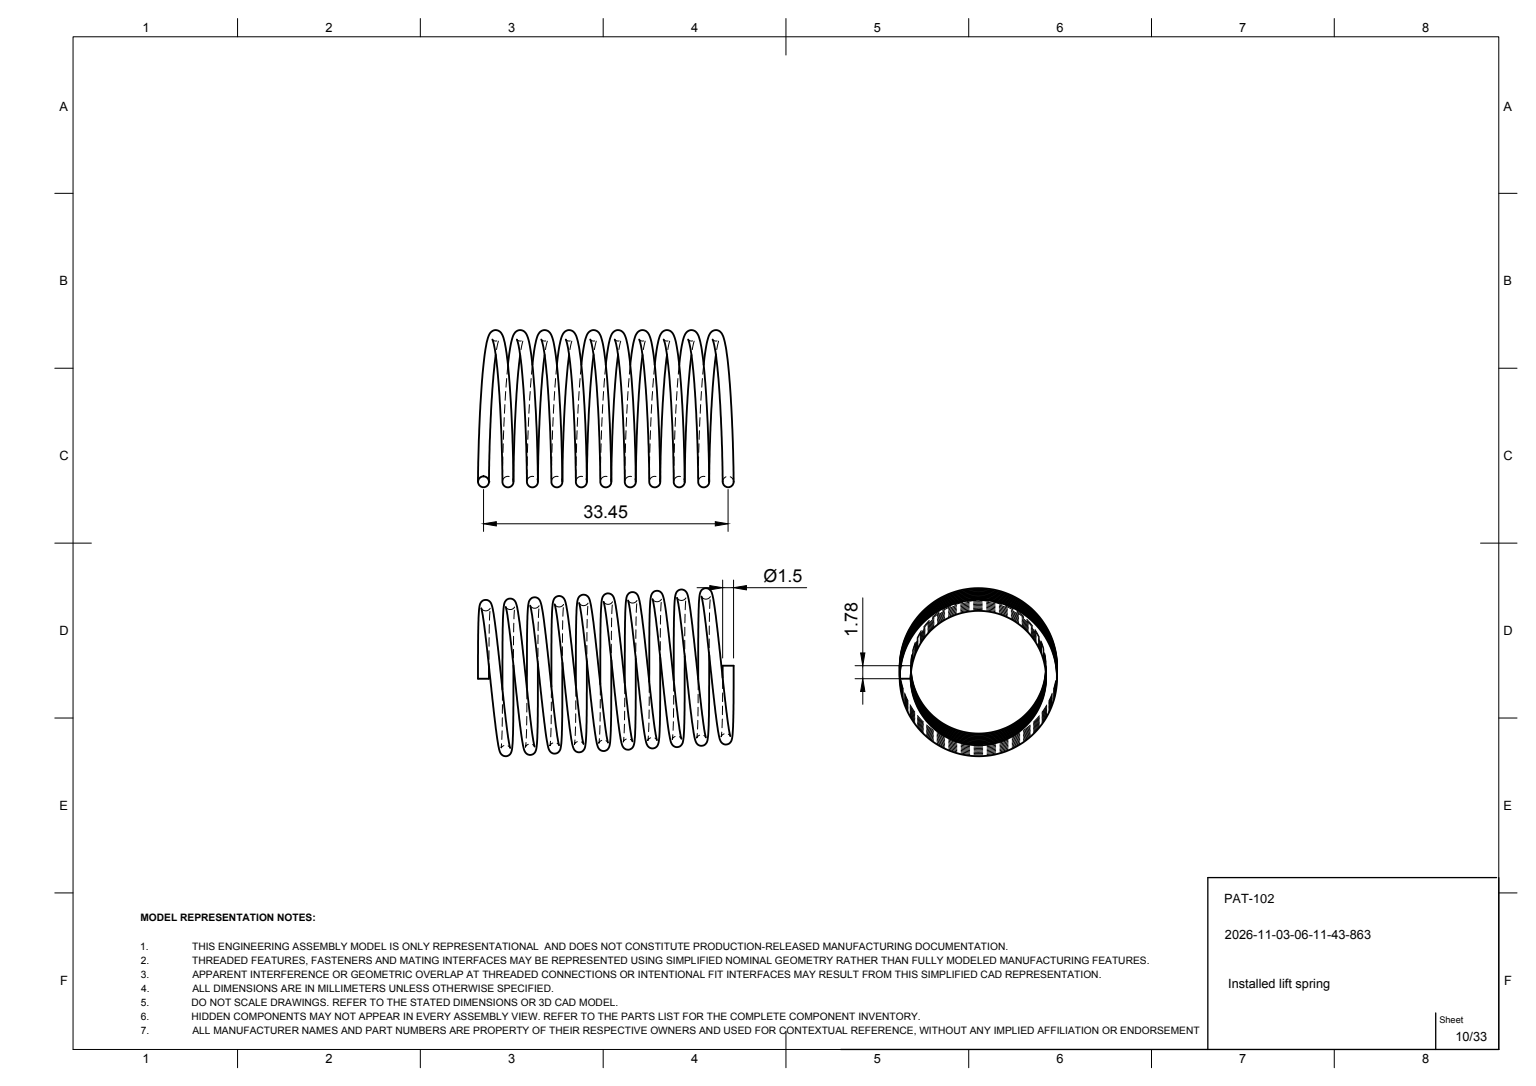
ISO-10303-21;
HEADER;
/* Generated by software containing ST-Developer
 * from STEP Tools, Inc. (www.steptools.com) 
 */

FILE_DESCRIPTION(
/* description */ ('Swing-away clamp arm'),
/* implementation_level */ '2;1');

FILE_NAME(
/* name */ 'Installed lift spring.step',
/* time_stamp */ '2026-10-28T03:26:03-07:00',
/* author */ (''),
/* organization */ (''),
/* preprocessor_version */ 'ST-DEVELOPER v20.2',
/* originating_system */ 'Autodesk Translation Framework v15.17.0.0',
/* authorisation */ '');

FILE_SCHEMA (('AUTOMOTIVE_DESIGN { 1 0 10303 214 3 1 1 }'));
ENDSEC;

DATA;
#10=MECHANICAL_DESIGN_GEOMETRIC_PRESENTATION_REPRESENTATION('',(#298),#10627);
#221=B_SPLINE_CURVE_WITH_KNOTS('',3,(#9145,#9146,#9147,#9148,#9149,#9150,
#9151,#9152,#9153,#9154,#9155,#9156,#9157,#9158,#9159,#9160,#9161,#9162,
#9163,#9164,#9165,#9166,#9167,#9168,#9169,#9170,#9171,#9172,#9173,#9174,
#9175,#9176,#9177,#9178,#9179,#9180,#9181,#9182,#9183,#9184,#9185,#9186,
#9187,#9188,#9189,#9190,#9191,#9192,#9193,#9194,#9195,#9196,#9197,#9198,
#9199,#9200,#9201,#9202,#9203,#9204,#9205,#9206,#9207,#9208,#9209,#9210,
#9211,#9212,#9213,#9214,#9215,#9216,#9217,#9218,#9219,#9220,#9221,#9222,
#9223,#9224,#9225,#9226,#9227,#9228,#9229,#9230,#9231,#9232,#9233,#9234,
#9235,#9236,#9237,#9238,#9239,#9240,#9241,#9242,#9243,#9244,#9245,#9246,
#9247,#9248,#9249,#9250,#9251,#9252,#9253,#9254,#9255,#9256,#9257,#9258,
#9259,#9260,#9261,#9262,#9263,#9264,#9265,#9266),.UNSPECIFIED.,.F.,.F.,
(4,1,1,1,1,1,1,1,1,1,1,1,1,1,1,1,1,1,1,1,1,1,1,1,1,1,1,1,1,1,1,1,1,1,1,
1,1,1,1,1,1,1,1,1,1,1,1,1,1,1,1,1,1,1,1,1,1,1,1,1,1,1,1,1,1,1,1,1,1,1,1,
1,1,1,1,1,1,1,1,1,1,1,1,1,1,1,1,1,1,1,1,1,1,1,1,1,1,1,1,1,1,1,1,1,1,1,1,
1,1,1,1,1,1,1,1,1,1,1,1,4),(0.,0.00892857142857143,0.0178571428571429,0.0267857142857143,
0.0357142857142857,0.0446428571428571,0.0535714285714286,0.0625,0.0714285714285714,
0.0803571428571428,0.0892857142857143,0.0982142857142857,0.107142857142857,
0.116071428571429,0.120535714285714,0.125,0.129464285714286,0.133928571428571,
0.138392857142857,0.142857142857143,0.150793650793651,0.154761904761905,
0.158730158730159,0.166666666666667,0.174603174603175,0.17989417989418,
0.19047619047619,0.198412698412698,0.206349206349206,0.214285714285714,
0.222222222222222,0.227513227513228,0.238095238095238,0.25,0.261904761904762,
0.273809523809524,0.285714285714286,0.297619047619048,0.30952380952381,
0.321428571428571,0.333333333333333,0.341269841269841,0.349206349206349,
0.357142857142857,0.365079365079365,0.37037037037037,0.380952380952381,
0.386243386243386,0.396825396825397,0.404761904761905,0.412698412698413,
0.420634920634921,0.428571428571429,0.44047619047619,0.452380952380952,
0.458333333333333,0.464285714285714,0.470238095238095,0.476190476190476,
0.484126984126984,0.492063492063492,0.5,0.502232142857143,0.504464285714286,
0.508928571428571,0.517857142857143,0.526785714285714,0.535714285714286,
0.544642857142857,0.553571428571429,0.5625,0.571428571428571,0.580357142857143,
0.589285714285714,0.598214285714286,0.607142857142857,0.616071428571429,
0.625,0.633928571428571,0.642857142857143,0.650793650793651,0.658730158730159,
0.666666666666667,0.678571428571428,0.69047619047619,0.702380952380952,
0.714285714285714,0.726190476190476,0.738095238095238,0.746031746031746,
0.753968253968254,0.761904761904762,0.76984126984127,0.777777777777778,
0.785714285714286,0.790178571428571,0.794642857142857,0.803571428571428,
0.8125,0.821428571428571,0.830357142857143,0.839285714285714,0.848214285714286,
0.857142857142857,0.866071428571429,0.875,0.883928571428571,0.892857142857143,
0.901785714285714,0.910714285714286,0.919642857142857,0.928571428571429,
0.9375,0.946428571428571,0.955357142857143,0.964285714285714,0.973214285714286,
0.982142857142857,0.991071428571429,1.),.UNSPECIFIED.);
#240=B_SPLINE_SURFACE_WITH_KNOTS('',3,3,((#7922,#7923,#7924,#7925,#7926,
#7927,#7928,#7929,#7930,#7931,#7932,#7933,#7934,#7935,#7936,#7937,#7938,
#7939,#7940,#7941,#7942,#7943,#7944,#7945,#7946,#7947,#7948,#7949,#7950,
#7951,#7952,#7953,#7954,#7955,#7956,#7957,#7958,#7959,#7960,#7961,#7962,
#7963,#7964,#7965,#7966,#7967,#7968,#7969,#7970,#7971,#7972,#7973,#7974,
#7975,#7976,#7977,#7978,#7979,#7980,#7981,#7982,#7983,#7984,#7985,#7986,
#7987,#7988,#7989,#7990,#7991,#7992,#7993,#7994,#7995,#7996,#7997,#7998,
#7999,#8000,#8001,#8002,#8003,#8004,#8005,#8006,#8007,#8008,#8009,#8010,
#8011,#8012,#8013,#8014,#8015,#8016,#8017,#8018,#8019,#8020,#8021,#8022,
#8023,#8024,#8025,#8026,#8027,#8028,#8029,#8030,#8031,#8032,#8033,#8034,
#8035,#8036,#8037,#8038,#8039,#8040,#8041,#8042,#8043),(#8044,#8045,#8046,
#8047,#8048,#8049,#8050,#8051,#8052,#8053,#8054,#8055,#8056,#8057,#8058,
#8059,#8060,#8061,#8062,#8063,#8064,#8065,#8066,#8067,#8068,#8069,#8070,
#8071,#8072,#8073,#8074,#8075,#8076,#8077,#8078,#8079,#8080,#8081,#8082,
#8083,#8084,#8085,#8086,#8087,#8088,#8089,#8090,#8091,#8092,#8093,#8094,
#8095,#8096,#8097,#8098,#8099,#8100,#8101,#8102,#8103,#8104,#8105,#8106,
#8107,#8108,#8109,#8110,#8111,#8112,#8113,#8114,#8115,#8116,#8117,#8118,
#8119,#8120,#8121,#8122,#8123,#8124,#8125,#8126,#8127,#8128,#8129,#8130,
#8131,#8132,#8133,#8134,#8135,#8136,#8137,#8138,#8139,#8140,#8141,#8142,
#8143,#8144,#8145,#8146,#8147,#8148,#8149,#8150,#8151,#8152,#8153,#8154,
#8155,#8156,#8157,#8158,#8159,#8160,#8161,#8162,#8163,#8164,#8165),(#8166,
#8167,#8168,#8169,#8170,#8171,#8172,#8173,#8174,#8175,#8176,#8177,#8178,
#8179,#8180,#8181,#8182,#8183,#8184,#8185,#8186,#8187,#8188,#8189,#8190,
#8191,#8192,#8193,#8194,#8195,#8196,#8197,#8198,#8199,#8200,#8201,#8202,
#8203,#8204,#8205,#8206,#8207,#8208,#8209,#8210,#8211,#8212,#8213,#8214,
#8215,#8216,#8217,#8218,#8219,#8220,#8221,#8222,#8223,#8224,#8225,#8226,
#8227,#8228,#8229,#8230,#8231,#8232,#8233,#8234,#8235,#8236,#8237,#8238,
#8239,#8240,#8241,#8242,#8243,#8244,#8245,#8246,#8247,#8248,#8249,#8250,
#8251,#8252,#8253,#8254,#8255,#8256,#8257,#8258,#8259,#8260,#8261,#8262,
#8263,#8264,#8265,#8266,#8267,#8268,#8269,#8270,#8271,#8272,#8273,#8274,
#8275,#8276,#8277,#8278,#8279,#8280,#8281,#8282,#8283,#8284,#8285,#8286,
#8287),(#8288,#8289,#8290,#8291,#8292,#8293,#8294,#8295,#8296,#8297,#8298,
#8299,#8300,#8301,#8302,#8303,#8304,#8305,#8306,#8307,#8308,#8309,#8310,
#8311,#8312,#8313,#8314,#8315,#8316,#8317,#8318,#8319,#8320,#8321,#8322,
#8323,#8324,#8325,#8326,#8327,#8328,#8329,#8330,#8331,#8332,#8333,#8334,
#8335,#8336,#8337,#8338,#8339,#8340,#8341,#8342,#8343,#8344,#8345,#8346,
#8347,#8348,#8349,#8350,#8351,#8352,#8353,#8354,#8355,#8356,#8357,#8358,
#8359,#8360,#8361,#8362,#8363,#8364,#8365,#8366,#8367,#8368,#8369,#8370,
#8371,#8372,#8373,#8374,#8375,#8376,#8377,#8378,#8379,#8380,#8381,#8382,
#8383,#8384,#8385,#8386,#8387,#8388,#8389,#8390,#8391,#8392,#8393,#8394,
#8395,#8396,#8397,#8398,#8399,#8400,#8401,#8402,#8403,#8404,#8405,#8406,
#8407,#8408,#8409),(#8410,#8411,#8412,#8413,#8414,#8415,#8416,#8417,#8418,
#8419,#8420,#8421,#8422,#8423,#8424,#8425,#8426,#8427,#8428,#8429,#8430,
#8431,#8432,#8433,#8434,#8435,#8436,#8437,#8438,#8439,#8440,#8441,#8442,
#8443,#8444,#8445,#8446,#8447,#8448,#8449,#8450,#8451,#8452,#8453,#8454,
#8455,#8456,#8457,#8458,#8459,#8460,#8461,#8462,#8463,#8464,#8465,#8466,
#8467,#8468,#8469,#8470,#8471,#8472,#8473,#8474,#8475,#8476,#8477,#8478,
#8479,#8480,#8481,#8482,#8483,#8484,#8485,#8486,#8487,#8488,#8489,#8490,
#8491,#8492,#8493,#8494,#8495,#8496,#8497,#8498,#8499,#8500,#8501,#8502,
#8503,#8504,#8505,#8506,#8507,#8508,#8509,#8510,#8511,#8512,#8513,#8514,
#8515,#8516,#8517,#8518,#8519,#8520,#8521,#8522,#8523,#8524,#8525,#8526,
#8527,#8528,#8529,#8530,#8531),(#8532,#8533,#8534,#8535,#8536,#8537,#8538,
#8539,#8540,#8541,#8542,#8543,#8544,#8545,#8546,#8547,#8548,#8549,#8550,
#8551,#8552,#8553,#8554,#8555,#8556,#8557,#8558,#8559,#8560,#8561,#8562,
#8563,#8564,#8565,#8566,#8567,#8568,#8569,#8570,#8571,#8572,#8573,#8574,
#8575,#8576,#8577,#8578,#8579,#8580,#8581,#8582,#8583,#8584,#8585,#8586,
#8587,#8588,#8589,#8590,#8591,#8592,#8593,#8594,#8595,#8596,#8597,#8598,
#8599,#8600,#8601,#8602,#8603,#8604,#8605,#8606,#8607,#8608,#8609,#8610,
#8611,#8612,#8613,#8614,#8615,#8616,#8617,#8618,#8619,#8620,#8621,#8622,
#8623,#8624,#8625,#8626,#8627,#8628,#8629,#8630,#8631,#8632,#8633,#8634,
#8635,#8636,#8637,#8638,#8639,#8640,#8641,#8642,#8643,#8644,#8645,#8646,
#8647,#8648,#8649,#8650,#8651,#8652,#8653),(#8654,#8655,#8656,#8657,#8658,
#8659,#8660,#8661,#8662,#8663,#8664,#8665,#8666,#8667,#8668,#8669,#8670,
#8671,#8672,#8673,#8674,#8675,#8676,#8677,#8678,#8679,#8680,#8681,#8682,
#8683,#8684,#8685,#8686,#8687,#8688,#8689,#8690,#8691,#8692,#8693,#8694,
#8695,#8696,#8697,#8698,#8699,#8700,#8701,#8702,#8703,#8704,#8705,#8706,
#8707,#8708,#8709,#8710,#8711,#8712,#8713,#8714,#8715,#8716,#8717,#8718,
#8719,#8720,#8721,#8722,#8723,#8724,#8725,#8726,#8727,#8728,#8729,#8730,
#8731,#8732,#8733,#8734,#8735,#8736,#8737,#8738,#8739,#8740,#8741,#8742,
#8743,#8744,#8745,#8746,#8747,#8748,#8749,#8750,#8751,#8752,#8753,#8754,
#8755,#8756,#8757,#8758,#8759,#8760,#8761,#8762,#8763,#8764,#8765,#8766,
#8767,#8768,#8769,#8770,#8771,#8772,#8773,#8774,#8775),(#8776,#8777,#8778,
#8779,#8780,#8781,#8782,#8783,#8784,#8785,#8786,#8787,#8788,#8789,#8790,
#8791,#8792,#8793,#8794,#8795,#8796,#8797,#8798,#8799,#8800,#8801,#8802,
#8803,#8804,#8805,#8806,#8807,#8808,#8809,#8810,#8811,#8812,#8813,#8814,
#8815,#8816,#8817,#8818,#8819,#8820,#8821,#8822,#8823,#8824,#8825,#8826,
#8827,#8828,#8829,#8830,#8831,#8832,#8833,#8834,#8835,#8836,#8837,#8838,
#8839,#8840,#8841,#8842,#8843,#8844,#8845,#8846,#8847,#8848,#8849,#8850,
#8851,#8852,#8853,#8854,#8855,#8856,#8857,#8858,#8859,#8860,#8861,#8862,
#8863,#8864,#8865,#8866,#8867,#8868,#8869,#8870,#8871,#8872,#8873,#8874,
#8875,#8876,#8877,#8878,#8879,#8880,#8881,#8882,#8883,#8884,#8885,#8886,
#8887,#8888,#8889,#8890,#8891,#8892,#8893,#8894,#8895,#8896,#8897),(#8898,
#8899,#8900,#8901,#8902,#8903,#8904,#8905,#8906,#8907,#8908,#8909,#8910,
#8911,#8912,#8913,#8914,#8915,#8916,#8917,#8918,#8919,#8920,#8921,#8922,
#8923,#8924,#8925,#8926,#8927,#8928,#8929,#8930,#8931,#8932,#8933,#8934,
#8935,#8936,#8937,#8938,#8939,#8940,#8941,#8942,#8943,#8944,#8945,#8946,
#8947,#8948,#8949,#8950,#8951,#8952,#8953,#8954,#8955,#8956,#8957,#8958,
#8959,#8960,#8961,#8962,#8963,#8964,#8965,#8966,#8967,#8968,#8969,#8970,
#8971,#8972,#8973,#8974,#8975,#8976,#8977,#8978,#8979,#8980,#8981,#8982,
#8983,#8984,#8985,#8986,#8987,#8988,#8989,#8990,#8991,#8992,#8993,#8994,
#8995,#8996,#8997,#8998,#8999,#9000,#9001,#9002,#9003,#9004,#9005,#9006,
#9007,#9008,#9009,#9010,#9011,#9012,#9013,#9014,#9015,#9016,#9017,#9018,
#9019),(#9020,#9021,#9022,#9023,#9024,#9025,#9026,#9027,#9028,#9029,#9030,
#9031,#9032,#9033,#9034,#9035,#9036,#9037,#9038,#9039,#9040,#9041,#9042,
#9043,#9044,#9045,#9046,#9047,#9048,#9049,#9050,#9051,#9052,#9053,#9054,
#9055,#9056,#9057,#9058,#9059,#9060,#9061,#9062,#9063,#9064,#9065,#9066,
#9067,#9068,#9069,#9070,#9071,#9072,#9073,#9074,#9075,#9076,#9077,#9078,
#9079,#9080,#9081,#9082,#9083,#9084,#9085,#9086,#9087,#9088,#9089,#9090,
#9091,#9092,#9093,#9094,#9095,#9096,#9097,#9098,#9099,#9100,#9101,#9102,
#9103,#9104,#9105,#9106,#9107,#9108,#9109,#9110,#9111,#9112,#9113,#9114,
#9115,#9116,#9117,#9118,#9119,#9120,#9121,#9122,#9123,#9124,#9125,#9126,
#9127,#9128,#9129,#9130,#9131,#9132,#9133,#9134,#9135,#9136,#9137,#9138,
#9139,#9140,#9141)),.UNSPECIFIED.,.T.,.F.,.F.,(4,1,1,1,1,1,1,4),(4,1,1,
1,1,1,1,1,1,1,1,1,1,1,1,1,1,1,1,1,1,1,1,1,1,1,1,1,1,1,1,1,1,1,1,1,1,1,1,
1,1,1,1,1,1,1,1,1,1,1,1,1,1,1,1,1,1,1,1,1,1,1,1,1,1,1,1,1,1,1,1,1,1,1,1,
1,1,1,1,1,1,1,1,1,1,1,1,1,1,1,1,1,1,1,1,1,1,1,1,1,1,1,1,1,1,1,1,1,1,1,1,
1,1,1,1,1,1,1,1,4),(-3.14159265358979,-2.24399475256414,-1.34639685153848,
-0.448798950512828,0.448798950512828,1.34639685153848,2.24399475256414,
3.14159265358979),(0.,0.00892857142857143,0.0178571428571429,0.0267857142857143,
0.0357142857142857,0.0446428571428571,0.0535714285714286,0.0625,0.0714285714285714,
0.0803571428571428,0.0892857142857143,0.0982142857142857,0.107142857142857,
0.116071428571429,0.120535714285714,0.125,0.129464285714286,0.133928571428571,
0.138392857142857,0.142857142857143,0.150793650793651,0.154761904761905,
0.158730158730159,0.166666666666667,0.174603174603175,0.17989417989418,
0.19047619047619,0.198412698412698,0.206349206349206,0.214285714285714,
0.222222222222222,0.227513227513228,0.238095238095238,0.25,0.261904761904762,
0.273809523809524,0.285714285714286,0.297619047619048,0.30952380952381,
0.321428571428571,0.333333333333333,0.341269841269841,0.349206349206349,
0.357142857142857,0.365079365079365,0.37037037037037,0.380952380952381,
0.386243386243386,0.396825396825397,0.404761904761905,0.412698412698413,
0.420634920634921,0.428571428571429,0.44047619047619,0.452380952380952,
0.458333333333333,0.464285714285714,0.470238095238095,0.476190476190476,
0.484126984126984,0.492063492063492,0.5,0.502232142857143,0.504464285714286,
0.508928571428571,0.517857142857143,0.526785714285714,0.535714285714286,
0.544642857142857,0.553571428571429,0.5625,0.571428571428571,0.580357142857143,
0.589285714285714,0.598214285714286,0.607142857142857,0.616071428571429,
0.625,0.633928571428571,0.642857142857143,0.650793650793651,0.658730158730159,
0.666666666666667,0.678571428571428,0.69047619047619,0.702380952380952,
0.714285714285714,0.726190476190476,0.738095238095238,0.746031746031746,
0.753968253968254,0.761904761904762,0.76984126984127,0.777777777777778,
0.785714285714286,0.790178571428571,0.794642857142857,0.803571428571428,
0.8125,0.821428571428571,0.830357142857143,0.839285714285714,0.848214285714286,
0.857142857142857,0.866071428571429,0.875,0.883928571428571,0.892857142857143,
0.901785714285714,0.910714285714286,0.919642857142857,0.928571428571429,
0.9375,0.946428571428571,0.955357142857143,0.964285714285714,0.973214285714286,
0.982142857142857,0.991071428571429,1.),.UNSPECIFIED.);
#246=SHAPE_REPRESENTATION_RELATIONSHIP('SRR','None',#10744,#272);
#272=ADVANCED_BREP_SHAPE_REPRESENTATION('',(#332),#10603);
#298=STYLED_ITEM('',(#10965),#332);
#332=MANIFOLD_SOLID_BREP('Body1',#4904);
#524=PLANE('',#5369);
#525=PLANE('',#5370);
#722=FACE_OUTER_BOUND('',#1055,.T.);
#723=FACE_OUTER_BOUND('',#1056,.T.);
#724=FACE_OUTER_BOUND('',#1057,.T.);
#1055=EDGE_LOOP('',(#3693,#3694,#3695,#3696));
#1056=EDGE_LOOP('',(#3697));
#1057=EDGE_LOOP('',(#3698));
#2046=CIRCLE('',#5367,0.075);
#2047=CIRCLE('',#5368,0.075);
#2399=VERTEX_POINT('',#9142);
#2400=VERTEX_POINT('',#9144);
#2879=EDGE_CURVE('',#2399,#2399,#2046,.T.);
#2880=EDGE_CURVE('',#2399,#2400,#221,.T.);
#2881=EDGE_CURVE('',#2400,#2400,#2047,.T.);
#3693=ORIENTED_EDGE('',*,*,#2879,.T.);
#3694=ORIENTED_EDGE('',*,*,#2880,.T.);
#3695=ORIENTED_EDGE('',*,*,#2881,.F.);
#3696=ORIENTED_EDGE('',*,*,#2880,.F.);
#3697=ORIENTED_EDGE('',*,*,#2881,.T.);
#3698=ORIENTED_EDGE('',*,*,#2879,.F.);
#4677=ADVANCED_FACE('',(#722),#240,.T.);
#4678=ADVANCED_FACE('',(#723),#524,.T.);
#4679=ADVANCED_FACE('',(#724),#525,.F.);
#4904=CLOSED_SHELL('',(#4677,#4678,#4679));
#5366=AXIS2_PLACEMENT_3D('',#7921,#6311,#6312);
#5367=AXIS2_PLACEMENT_3D('',#9143,#6313,#6314);
#5368=AXIS2_PLACEMENT_3D('',#9267,#6315,#6316);
#5369=AXIS2_PLACEMENT_3D('',#9268,#6317,#6318);
#5370=AXIS2_PLACEMENT_3D('',#9269,#6319,#6320);
#6311=DIRECTION('axis',(0.,0.,1.));
#6312=DIRECTION('refdir',(1.,0.,0.));
#6313=DIRECTION('center_axis',(-0.000134431341915714,0.998590099522227,
0.0530829074599677));
#6314=DIRECTION('ref_axis',(7.14608168190195E-6,-0.0530829069789608,0.998590108570877));
#6315=DIRECTION('center_axis',(0.000134431323893231,0.998590099521685,0.0530829074702145));
#6316=DIRECTION('ref_axis',(0.202244098525442,0.0519588076800388,-0.977955830759294));
#6317=DIRECTION('center_axis',(0.000134431323893231,0.998590099521685,0.0530829074702145));
#6318=DIRECTION('ref_axis',(0.202244098525442,0.0519588076800388,-0.977955830759294));
#6319=DIRECTION('center_axis',(-0.000134431341915714,0.998590099522227,
0.0530829074599677));
#6320=DIRECTION('ref_axis',(7.14608168190194E-6,-0.0530829069789608,0.998590108570877));
#7921=CARTESIAN_POINT('',(0.,0.,0.));
#7922=CARTESIAN_POINT('Ctrl Pts',(0.999999464043874,0.00398121802342207,
2.00010574185718));
#7923=CARTESIAN_POINT('Ctrl Pts',(0.999974206061282,0.19160391813607,2.01007936209659));
#7924=CARTESIAN_POINT('Ctrl Pts',(0.892358674149497,0.565284907029969,2.03003975780563));
#7925=CARTESIAN_POINT('Ctrl Pts',(0.455908354460267,0.955754980387012,2.06005123671475));
#7926=CARTESIAN_POINT('Ctrl Pts',(-0.122563158588718,1.05404138225222,2.09012808179557));
#7927=CARTESIAN_POINT('Ctrl Pts',(-0.665982422429721,0.829161410069987,
2.12027227517451));
#7928=CARTESIAN_POINT('Ctrl Pts',(-1.00720268117277,0.348508238874394,2.15048257508427));
#7929=CARTESIAN_POINT('Ctrl Pts',(-1.04050120808252,-0.241264621011279,
2.18075912672908));
#7930=CARTESIAN_POINT('Ctrl Pts',(-0.754298406118339,-0.759496345182109,
2.21110138862918));
#7931=CARTESIAN_POINT('Ctrl Pts',(-0.235139085598783,-1.04662471701868,
2.24150905560043));
#7932=CARTESIAN_POINT('Ctrl Pts',(0.358466657407177,-1.0134893307861,2.27198163744466));
#7933=CARTESIAN_POINT('Ctrl Pts',(0.844481314225998,-0.668830870873697,
2.30251864881201));
#7934=CARTESIAN_POINT('Ctrl Pts',(1.07309171546203,-0.117397710656463,2.33311952120739));
#7935=CARTESIAN_POINT('Ctrl Pts',(0.973085863935879,0.472631726678538,2.36378364003101));
#7936=CARTESIAN_POINT('Ctrl Pts',(0.640186615940372,0.844850208282888,2.38938921676183));
#7937=CARTESIAN_POINT('Ctrl Pts',(0.285207254948024,1.00321211946817,2.40990460122644));
#7938=CARTESIAN_POINT('Ctrl Pts',(-0.00357278466147455,1.04413748919053,
2.42530650345941));
#7939=CARTESIAN_POINT('Ctrl Pts',(-0.292753333069628,1.00327492007872,2.4407236705559));
#7940=CARTESIAN_POINT('Ctrl Pts',(-0.559610149845377,0.883939984413932,
2.45615599894115));
#7941=CARTESIAN_POINT('Ctrl Pts',(-0.783072629292576,0.695150535469123,
2.47160338259101));
#7942=CARTESIAN_POINT('Ctrl Pts',(-0.9883155178948,0.388599518613216,2.49107446360262));
#7943=CARTESIAN_POINT('Ctrl Pts',(-1.06097928852007,0.0299698265249316,
2.50999804459158));
#7944=CARTESIAN_POINT('Ctrl Pts',(-1.00026874085688,-0.31207309433285,2.52837129391011));
#7945=CARTESIAN_POINT('Ctrl Pts',(-0.85772117693898,-0.628943233787528,
2.54675983289627));
#7946=CARTESIAN_POINT('Ctrl Pts',(-0.539023756454129,-0.940248430945502,
2.56977396086322));
#7947=CARTESIAN_POINT('Ctrl Pts',(-0.0813539710712336,-1.06875629404709,
2.59436218564022));
#7948=CARTESIAN_POINT('Ctrl Pts',(0.440709506996878,-0.995074461032676,
2.6220606386953));
#7949=CARTESIAN_POINT('Ctrl Pts',(0.881652173543376,-0.668351901468915,
2.64980261114177));
#7950=CARTESIAN_POINT('Ctrl Pts',(1.0852948664173,-0.105373203004237,2.68068203601616));
#7951=CARTESIAN_POINT('Ctrl Pts',(1.00539530848997,0.426480980519131,2.70851510392812));
#7952=CARTESIAN_POINT('Ctrl Pts',(0.679609573339881,0.857002336026301,2.7363888804944));
#7953=CARTESIAN_POINT('Ctrl Pts',(0.242228396206659,1.05406947259606,2.76120094819001));
#7954=CARTESIAN_POINT('Ctrl Pts',(-0.289433825273236,1.05900157503401,2.78914691397882));
#7955=CARTESIAN_POINT('Ctrl Pts',(-0.861030373991185,0.756502517113054,
2.82179513727801));
#7956=CARTESIAN_POINT('Ctrl Pts',(-1.15948386741598,-0.00245881106342116,
2.8622922968233));
#7957=CARTESIAN_POINT('Ctrl Pts',(-0.849819252545902,-0.791606149879273,
2.9044266522989));
#7958=CARTESIAN_POINT('Ctrl Pts',(-0.0848273064559805,-1.16047682132822,
2.94663705560064));
#7959=CARTESIAN_POINT('Ctrl Pts',(0.728338616139595,-0.909963609903424,
2.98891980674896));
#7960=CARTESIAN_POINT('Ctrl Pts',(1.15452570093491,-0.172022292800125,3.03127110274204));
#7961=CARTESIAN_POINT('Ctrl Pts',(0.965079959728901,0.659906484623926,3.07368702284038));
#7962=CARTESIAN_POINT('Ctrl Pts',(0.258512451458961,1.14196808324737,3.11616354351132));
#7963=CARTESIAN_POINT('Ctrl Pts',(-0.492717397384934,1.02781794268986,3.15397066853381));
#7964=CARTESIAN_POINT('Ctrl Pts',(-0.950847731766782,0.578891230696036,
3.18708578741999));
#7965=CARTESIAN_POINT('Ctrl Pts',(-1.11322603418831,0.0543699563964829,
3.21549214280387));
#7966=CARTESIAN_POINT('Ctrl Pts',(-1.00397682800075,-0.485299668185688,
3.24391918371992));
#7967=CARTESIAN_POINT('Ctrl Pts',(-0.689560596566738,-0.85912025786842,
3.2692049003822));
#7968=CARTESIAN_POINT('Ctrl Pts',(-0.203462101275883,-1.09903917913844,
3.29766639858301));
#7969=CARTESIAN_POINT('Ctrl Pts',(0.296274556510708,-1.07870085350966,3.32298079518316));
#7970=CARTESIAN_POINT('Ctrl Pts',(0.813909810244539,-0.768416856681802,
3.35464092662437));
#7971=CARTESIAN_POINT('Ctrl Pts',(1.10016251506307,-0.282678926353398,3.38314956983213));
#7972=CARTESIAN_POINT('Ctrl Pts',(1.06842542005047,0.330699838209083,3.41484232929802));
#7973=CARTESIAN_POINT('Ctrl Pts',(0.781036889262004,0.801635745996559,3.44337716794684));
#7974=CARTESIAN_POINT('Ctrl Pts',(0.3026681656048,1.07751158150631,3.47192198965488));
#7975=CARTESIAN_POINT('Ctrl Pts',(-0.341977208139237,1.09513778685306,3.5052343169007));
#7976=CARTESIAN_POINT('Ctrl Pts',(-0.975597618652369,0.664760099314692,
3.54331757606612));
#7977=CARTESIAN_POINT('Ctrl Pts',(-1.13429370842399,-0.0357778387848846,
3.57903024860792));
#7978=CARTESIAN_POINT('Ctrl Pts',(-0.952497172320662,-0.550291907933128,
3.60760379990449));
#7979=CARTESIAN_POINT('Ctrl Pts',(-0.68624513734708,-0.860512981218381,
3.62903507783467));
#7980=CARTESIAN_POINT('Ctrl Pts',(-0.324306798008731,-1.0514860754467,3.65046688028005));
#7981=CARTESIAN_POINT('Ctrl Pts',(0.127344232453658,-1.10276625857497,3.674279919598));
#7982=CARTESIAN_POINT('Ctrl Pts',(0.607784221866902,-0.941400265606059,
3.70047332316486));
#7983=CARTESIAN_POINT('Ctrl Pts',(0.983690388895233,-0.535896868540009,
3.72904537472281));
#7984=CARTESIAN_POINT('Ctrl Pts',(1.08731538430027,-0.128732018548745,3.75076902067426));
#7985=CARTESIAN_POINT('Ctrl Pts',(1.06753777509939,0.150334725456009,3.7656464393213));
#7986=CARTESIAN_POINT('Ctrl Pts',(1.02549367550628,0.347236435696266,3.7763575734054));
#7987=CARTESIAN_POINT('Ctrl Pts',(0.880884191480398,0.671592660752369,3.7951003560531));
#7988=CARTESIAN_POINT('Ctrl Pts',(0.491799935626419,1.0196644890383,3.82187027476111));
#7989=CARTESIAN_POINT('Ctrl Pts',(-0.126065746592581,1.12455786056488,3.85398342973913));
#7990=CARTESIAN_POINT('Ctrl Pts',(-0.704583522010695,0.88486307777345,3.88608387297236));
#7991=CARTESIAN_POINT('Ctrl Pts',(-1.06683466983354,0.3742832244399,3.91816964977168));
#7992=CARTESIAN_POINT('Ctrl Pts',(-1.10184933977514,-0.250419432627018,
3.95023881727803));
#7993=CARTESIAN_POINT('Ctrl Pts',(-0.799326718711519,-0.797694380880393,
3.98228945733906));
#7994=CARTESIAN_POINT('Ctrl Pts',(-0.252343111177166,-1.09993153075449,
4.01431965364637));
#7995=CARTESIAN_POINT('Ctrl Pts',(0.371159169345164,-1.06485412373635,4.0463275194738));
#7996=CARTESIAN_POINT('Ctrl Pts',(0.880047504125487,-0.703696890362346,
4.07831118189475));
#7997=CARTESIAN_POINT('Ctrl Pts',(1.11857837754389,-0.127626743256515,4.11026879475596));
#7998=CARTESIAN_POINT('Ctrl Pts',(1.01416153614381,0.486524030990474,4.14219853012843));
#7999=CARTESIAN_POINT('Ctrl Pts',(0.599338058827864,0.950520440175857,4.17409858361638));
#8000=CARTESIAN_POINT('Ctrl Pts',(0.00190308953361062,1.12257447034417,
4.20596718959497));
#8001=CARTESIAN_POINT('Ctrl Pts',(-0.595087816877256,0.950429978912684,
4.23780259148061));
#8002=CARTESIAN_POINT('Ctrl Pts',(-0.992818074176864,0.504960206465758,
4.26842528448615));
#8003=CARTESIAN_POINT('Ctrl Pts',(-1.10558192615926,-0.0535255134762696,
4.29783816996833));
#8004=CARTESIAN_POINT('Ctrl Pts',(-0.944245633155887,-0.574182433998452,
4.326044460862));
#8005=CARTESIAN_POINT('Ctrl Pts',(-0.489615552103502,-1.02023046107543,
4.35891537170686));
#8006=CARTESIAN_POINT('Ctrl Pts',(0.255873406558148,-1.13223620757883,4.39642822383059));
#8007=CARTESIAN_POINT('Ctrl Pts',(0.956585537399415,-0.654531370431507,
4.43855371945495));
#8008=CARTESIAN_POINT('Ctrl Pts',(1.14416456861692,0.170066871142059,4.48059920430672));
#8009=CARTESIAN_POINT('Ctrl Pts',(0.722117099067864,0.901002181388938,4.52256123999552));
#8010=CARTESIAN_POINT('Ctrl Pts',(-0.0838676738781217,1.14921441407926,
4.5644365266184));
#8011=CARTESIAN_POINT('Ctrl Pts',(-0.755677502986392,0.824069849946143,
4.60157908243497));
#8012=CARTESIAN_POINT('Ctrl Pts',(-1.05498104408691,0.271521112381307,4.63401858831428));
#8013=CARTESIAN_POINT('Ctrl Pts',(-1.05483403133078,-0.26522135570406,4.66178172056988));
#8014=CARTESIAN_POINT('Ctrl Pts',(-0.79840547489227,-0.736599185468657,
4.68950186792131));
#8015=CARTESIAN_POINT('Ctrl Pts',(-0.3483499377511,-1.02663834291108,4.71717822726345));
#8016=CARTESIAN_POINT('Ctrl Pts',(0.184757632451299,-1.06688722115596,4.74481003558103));
#8017=CARTESIAN_POINT('Ctrl Pts',(0.600256695779753,-0.878980608467174,
4.7683735201888));
#8018=CARTESIAN_POINT('Ctrl Pts',(0.853850233649786,-0.610120445383555,
4.78788851920089));
#8019=CARTESIAN_POINT('Ctrl Pts',(1.03381570897682,-0.262894148472765,4.80853189587555));
#8020=CARTESIAN_POINT('Ctrl Pts',(1.06215687349528,0.238874309450968,4.83429913779336));
#8021=CARTESIAN_POINT('Ctrl Pts',(0.770634803840811,0.765869068483215,4.86515976481244));
#8022=CARTESIAN_POINT('Ctrl Pts',(0.244684747552399,1.05635550605388,4.89595947659513));
#8023=CARTESIAN_POINT('Ctrl Pts',(-0.354100647382748,1.02257824395859,4.92669748292077));
#8024=CARTESIAN_POINT('Ctrl Pts',(-0.842095960257555,0.676096127224308,
4.95737304397893));
#8025=CARTESIAN_POINT('Ctrl Pts',(-1.07050216965279,0.124232350128257,4.98798547954758));
#8026=CARTESIAN_POINT('Ctrl Pts',(-0.970487698233666,-0.463339790807337,
5.01853416178037));
#8027=CARTESIAN_POINT('Ctrl Pts',(-0.57403535125674,-0.906703305752076,
5.04901852189829));
#8028=CARTESIAN_POINT('Ctrl Pts',(-0.00367933936324437,-1.07083384017741,
5.07943804916124));
#8029=CARTESIAN_POINT('Ctrl Pts',(0.56535226719551,-0.906710964597204,5.10979228847672));
#8030=CARTESIAN_POINT('Ctrl Pts',(0.95899197878984,-0.465956326824321,5.14008084401914));
#8031=CARTESIAN_POINT('Ctrl Pts',(1.05758360680831,0.115400410376887,5.17030337915801));
#8032=CARTESIAN_POINT('Ctrl Pts',(0.832257130959616,0.658907139635372,5.20045961311858));
#8033=CARTESIAN_POINT('Ctrl Pts',(0.353362036446966,0.998475173781019,5.23054933034559));
#8034=CARTESIAN_POINT('Ctrl Pts',(-0.231493376683462,1.03113233690688,5.26057235733975));
#8035=CARTESIAN_POINT('Ctrl Pts',(-0.742941371583914,0.748253733713579,
5.29052861685377));
#8036=CARTESIAN_POINT('Ctrl Pts',(-1.02486870130036,0.23775759542928,5.3204180022368));
#8037=CARTESIAN_POINT('Ctrl Pts',(-0.992064317380329,-0.343173817499407,
5.3502406538254));
#8038=CARTESIAN_POINT('Ctrl Pts',(-0.655975229859479,-0.81659286891466,
5.37999633599993));
#8039=CARTESIAN_POINT('Ctrl Pts',(-0.120753665413257,-1.03807600951265,
5.40968580999697));
#8040=CARTESIAN_POINT('Ctrl Pts',(0.44897427078276,-0.941278849111864,5.43930775328404));
#8041=CARTESIAN_POINT('Ctrl Pts',(0.878820594563222,-0.556707495126734,
5.46886560818098));
#8042=CARTESIAN_POINT('Ctrl Pts',(0.984806813297395,-0.188706783169536,
5.48852259094232));
#8043=CARTESIAN_POINT('Ctrl Pts',(0.984831692610592,-0.00389691057600537,
5.49834668730695));
#8044=CARTESIAN_POINT('Ctrl Pts',(0.97755951672157,0.00397819713203481,
2.00010574185718));
#8045=CARTESIAN_POINT('Ctrl Pts',(0.977534817777559,0.1874482168994,2.009858614518));
#8046=CARTESIAN_POINT('Ctrl Pts',(0.872339507129369,0.552742035957965,2.02937002260745));
#8047=CARTESIAN_POINT('Ctrl Pts',(0.445612976498857,0.934542787186617,2.05871357126365));
#8048=CARTESIAN_POINT('Ctrl Pts',(-0.120030718543652,1.03065208177895,2.08812225036493));
#8049=CARTESIAN_POINT('Ctrl Pts',(-0.651468641058004,0.81074656763505,2.11760084182634));
#8050=CARTESIAN_POINT('Ctrl Pts',(-0.985218541716035,0.340638135385857,
2.14714764844481));
#8051=CARTESIAN_POINT('Ctrl Pts',(-1.01780770850236,-0.236290452249486,
2.1767638465366));
#8052=CARTESIAN_POINT('Ctrl Pts',(-0.737804384439041,-0.743333134894278,
2.20644924954275));
#8053=CARTESIAN_POINT('Ctrl Pts',(-0.229775908433837,-1.02432739723473,
2.23620424753441));
#8054=CARTESIAN_POINT('Ctrl Pts',(0.351236203556259,-0.991916639617009,
2.26602880347846));
#8055=CARTESIAN_POINT('Ctrl Pts',(0.827059185578202,-0.654513807733518,
2.29592316173363));
#8056=CARTESIAN_POINT('Ctrl Pts',(1.05094913773538,-0.114539223746344,2.32588691927782));
#8057=CARTESIAN_POINT('Ctrl Pts',(0.953019218248555,0.463396416555815,2.35592076218885));
#8058=CARTESIAN_POINT('Ctrl Pts',(0.626882081793141,0.828092290475244,2.3810056356548));
#8059=CARTESIAN_POINT('Ctrl Pts',(0.279001515164431,0.98329371752799,2.40111022029383));
#8060=CARTESIAN_POINT('Ctrl Pts',(-0.00404384991316098,1.02341077763893,
2.41620568810213));
#8061=CARTESIAN_POINT('Ctrl Pts',(-0.287527493131225,0.983358922547369,
2.43131843531318));
#8062=CARTESIAN_POINT('Ctrl Pts',(-0.549169823355069,0.866360638694792,
2.44644850402512));
#8063=CARTESIAN_POINT('Ctrl Pts',(-0.768302851844728,0.681237070886304,
2.46159552744086));
#8064=CARTESIAN_POINT('Ctrl Pts',(-0.969606942749099,0.380577490179153,
2.48069205537781));
#8065=CARTESIAN_POINT('Ctrl Pts',(-1.04090110132001,0.0287889134734739,
2.49925258741977));
#8066=CARTESIAN_POINT('Ctrl Pts',(-0.981332549271593,-0.306846625190479,
2.51728108741502));
#8067=CARTESIAN_POINT('Ctrl Pts',(-0.841439122236331,-0.617828920196817,
2.53532696806566));
#8068=CARTESIAN_POINT('Ctrl Pts',(-0.528617679054796,-0.923413568511115,
2.55791563566096));
#8069=CARTESIAN_POINT('Ctrl Pts',(-0.0792029712632743,-1.04963369664941,
2.5820592733512));
#8070=CARTESIAN_POINT('Ctrl Pts',(0.433613375636684,-0.977259413861191,
2.60926626333433));
#8071=CARTESIAN_POINT('Ctrl Pts',(0.86691020025717,-0.656268692809005,2.63652289720304));
#8072=CARTESIAN_POINT('Ctrl Pts',(1.06712276644286,-0.102855375409246,2.66687533427124));
#8073=CARTESIAN_POINT('Ctrl Pts',(0.98857794766632,0.420176175347904,2.69424420831848));
#8074=CARTESIAN_POINT('Ctrl Pts',(0.668088783928289,0.84372911958199,2.72166407525147));
#8075=CARTESIAN_POINT('Ctrl Pts',(0.237626170167846,1.03771059246847,2.74608285338797));
#8076=CARTESIAN_POINT('Ctrl Pts',(-0.285834074724791,1.0425713500964,2.77359680577556));
#8077=CARTESIAN_POINT('Ctrl Pts',(-0.848855562512735,0.744685054006121,
2.80575161465571));
#8078=CARTESIAN_POINT('Ctrl Pts',(-1.14307267505854,-0.00325442246706518,
2.8456576200506));
#8079=CARTESIAN_POINT('Ctrl Pts',(-0.837781318697799,-0.781552909693705,
2.88720708486476));
#8080=CARTESIAN_POINT('Ctrl Pts',(-0.0828721428173334,-1.14567971574881,
2.92885934862034));
#8081=CARTESIAN_POINT('Ctrl Pts',(0.720219591828141,-0.898389153408221,
2.97061256607032));
#8082=CARTESIAN_POINT('Ctrl Pts',(1.14151252862521,-0.169156474837318,3.01246340210315));
#8083=CARTESIAN_POINT('Ctrl Pts',(0.954270451079617,0.653649229724285,3.05440814190739));
#8084=CARTESIAN_POINT('Ctrl Pts',(0.255025659690968,1.13086513577111,3.09644483636185));
#8085=CARTESIAN_POINT('Ctrl Pts',(-0.489061511145333,1.01792230474927,3.1338859178981));
#8086=CARTESIAN_POINT('Ctrl Pts',(-0.943166447988804,0.572999920918024,
3.1667058728693));
#8087=CARTESIAN_POINT('Ctrl Pts',(-1.10422957591935,0.0528956969736171,
3.19486998840399));
#8088=CARTESIAN_POINT('Ctrl Pts',(-0.99585841718268,-0.482570482219919,
3.22307483505779));
#8089=CARTESIAN_POINT('Ctrl Pts',(-0.68379925456048,-0.853657824468507,
3.24816978426164));
#8090=CARTESIAN_POINT('Ctrl Pts',(-0.201021562509179,-1.09194860971787,
3.27643689660237));
#8091=CARTESIAN_POINT('Ctrl Pts',(0.295507073604264,-1.07180490446086,3.3015851015371));
#8092=CARTESIAN_POINT('Ctrl Pts',(0.810140242218131,-0.763341809894584,
3.33305898227309));
#8093=CARTESIAN_POINT('Ctrl Pts',(1.09493646689165,-0.280204938812027,3.36141446000882));
#8094=CARTESIAN_POINT('Ctrl Pts',(1.06338198271354,0.330333565929847,3.39295813889907));
#8095=CARTESIAN_POINT('Ctrl Pts',(0.777210322504459,0.799346590189962,3.42137245074107));
#8096=CARTESIAN_POINT('Ctrl Pts',(0.300565645225493,1.0742632068725,3.44981223300455));
#8097=CARTESIAN_POINT('Ctrl Pts',(-0.342137134487029,1.09188368707827,3.48302128705105));
#8098=CARTESIAN_POINT('Ctrl Pts',(-0.974318785413307,0.662612446779102,
3.52100929419482));
#8099=CARTESIAN_POINT('Ctrl Pts',(-1.13288648807811,-0.0368107892008958,
3.55666065886606));
#8100=CARTESIAN_POINT('Ctrl Pts',(-0.951263764107293,-0.550894470418624,
3.58520750931815));
#8101=CARTESIAN_POINT('Ctrl Pts',(-0.685143524722543,-0.860992717462809,
3.60662854664387));
#8102=CARTESIAN_POINT('Ctrl Pts',(-0.323240816819056,-1.05196957863857,
3.62805661151224));
#8103=CARTESIAN_POINT('Ctrl Pts',(0.128560007356371,-1.10328952951889,3.65187603774534));
#8104=CARTESIAN_POINT('Ctrl Pts',(0.609407280723653,-0.941828387728985,
3.67808837863482));
#8105=CARTESIAN_POINT('Ctrl Pts',(0.98586930660155,-0.535768218197723,3.70670010871054));
#8106=CARTESIAN_POINT('Ctrl Pts',(1.0897063480334,-0.127854204552833,3.72846073180296));
#8107=CARTESIAN_POINT('Ctrl Pts',(1.06988164984646,0.15186778414323,3.74337260693928));
#8108=CARTESIAN_POINT('Ctrl Pts',(1.02773317276792,0.34926212253662,3.75411020888856));
#8109=CARTESIAN_POINT('Ctrl Pts',(0.882741007204007,0.674496884799054,3.77290255357357));
#8110=CARTESIAN_POINT('Ctrl Pts',(0.492481996563103,1.02367766444837,3.79975197771051));
#8111=CARTESIAN_POINT('Ctrl Pts',(-0.127690565781102,1.12901692327556,3.8319825979689));
#8112=CARTESIAN_POINT('Ctrl Pts',(-0.708748153845812,0.888319810350649,
3.86421960143728));
#8113=CARTESIAN_POINT('Ctrl Pts',(-1.07284204822087,0.37523040851078,3.89646195079746));
#8114=CARTESIAN_POINT('Ctrl Pts',(-1.10810231534743,-0.252955497845161,
3.92870698364651));
#8115=CARTESIAN_POINT('Ctrl Pts',(-0.803754630503077,-0.803637553165077,
3.96095281863656));
#8116=CARTESIAN_POINT('Ctrl Pts',(-0.253088561756074,-1.10796766192506,
3.99319723942644));
#8117=CARTESIAN_POINT('Ctrl Pts',(0.375010957528947,-1.07268207150159,4.02543819894899));
#8118=CARTESIAN_POINT('Ctrl Pts',(0.887976540139475,-0.708692354908092,
4.05767359098646));
#8119=CARTESIAN_POINT('Ctrl Pts',(1.12858897297226,-0.127723402477217,4.08990133451333));
#8120=CARTESIAN_POINT('Ctrl Pts',(1.02326898300414,0.492031189427128,4.12211937335469));
#8121=CARTESIAN_POINT('Ctrl Pts',(0.604466062779254,0.960551404367795,4.15432557540022));
#8122=CARTESIAN_POINT('Ctrl Pts',(0.000927783036573728,1.13441322120194,
4.18651801173377));
#8123=CARTESIAN_POINT('Ctrl Pts',(-0.602520120716071,0.960458611226862,
4.21869431046299));
#8124=CARTESIAN_POINT('Ctrl Pts',(-1.00478741507514,0.509967747015279,4.24966196687484));
#8125=CARTESIAN_POINT('Ctrl Pts',(-1.11892334048673,-0.0551203638852278,
4.27942038227802));
#8126=CARTESIAN_POINT('Ctrl Pts',(-0.955613823551837,-0.582210419872125,
4.30797396885712));
#8127=CARTESIAN_POINT('Ctrl Pts',(-0.495204396789493,-1.03399629100515,
4.34126381542087));
#8128=CARTESIAN_POINT('Ctrl Pts',(0.2602289300512,-1.14757077870588,4.37927522482165));
#8129=CARTESIAN_POINT('Ctrl Pts',(0.970816206161694,-0.663265764508169,
4.42198822284881));
#8130=CARTESIAN_POINT('Ctrl Pts',(1.1612353098011,0.173412559077483,4.46464709152681));
#8131=CARTESIAN_POINT('Ctrl Pts',(0.73281467250382,0.915574596057104,4.50724834203436));
#8132=CARTESIAN_POINT('Ctrl Pts',(-0.085964988811639,1.16782799270487,4.54978699118941));
#8133=CARTESIAN_POINT('Ctrl Pts',(-0.768880602583059,0.837392966288513,
4.58753928679426));
#8134=CARTESIAN_POINT('Ctrl Pts',(-1.07329276575036,0.275486454169533,4.62052734960056));
#8135=CARTESIAN_POINT('Ctrl Pts',(-1.07316083376288,-0.27056471925353,4.64877133408048));
#8136=CARTESIAN_POINT('Ctrl Pts',(-0.812223242657351,-0.750291341226326,
4.67698085025682));
#8137=CARTESIAN_POINT('Ctrl Pts',(-0.354063516147758,-1.04557309377014,
4.70515509535978));
#8138=CARTESIAN_POINT('Ctrl Pts',(0.188835848046625,-1.08658576479028,4.73329424506581));
#8139=CARTESIAN_POINT('Ctrl Pts',(0.612091477193082,-0.89518184092728,4.75729595235333));
#8140=CARTESIAN_POINT('Ctrl Pts',(0.87049090381391,-0.621232336099561,4.77718028775068));
#8141=CARTESIAN_POINT('Ctrl Pts',(1.05389711917837,-0.267373370743659,4.79821770027757));
#8142=CARTESIAN_POINT('Ctrl Pts',(1.0828048480663,0.2440947028953,4.82448212353492));
#8143=CARTESIAN_POINT('Ctrl Pts',(0.785570688143936,0.781464268917798,4.85594880718113));
#8144=CARTESIAN_POINT('Ctrl Pts',(0.249128587108361,1.07776823295182,4.88736261138121));
#8145=CARTESIAN_POINT('Ctrl Pts',(-0.361785836370703,1.04332703153431,4.91872252432293));
#8146=CARTESIAN_POINT('Ctrl Pts',(-0.859808049698745,0.689748559723978,
4.95002707792092));
#8147=CARTESIAN_POINT('Ctrl Pts',(-1.09297615308804,0.126424919553853,4.98127509388506));
#8148=CARTESIAN_POINT('Ctrl Pts',(-0.990875767219502,-0.47349721224129,
5.0124653393971));
#8149=CARTESIAN_POINT('Ctrl Pts',(-0.586016424119173,-0.926284211843029,
5.04359668436538));
#8150=CARTESIAN_POINT('Ctrl Pts',(-0.00343903085660042,-1.09394513826332,
5.07466803457235));
#8151=CARTESIAN_POINT('Ctrl Pts',(0.57789653224993,-0.926285315052589,5.10567835345191));
#8152=CARTESIAN_POINT('Ctrl Pts',(0.9801178138107,-0.475936671342823,5.13662665912829));
#8153=CARTESIAN_POINT('Ctrl Pts',(1.08087952050974,0.118166939826646,5.16751202559587));
#8154=CARTESIAN_POINT('Ctrl Pts',(0.850589387397783,0.673663880453797,5.19833358312002));
#8155=CARTESIAN_POINT('Ctrl Pts',(0.361082693325379,1.02076245584766,5.22909051751435));
#8156=CARTESIAN_POINT('Ctrl Pts',(-0.236787832380174,1.05414991601765,5.2597820690211));
#8157=CARTESIAN_POINT('Ctrl Pts',(-0.759654102884898,0.764957789837657,
5.29040754589614));
#8158=CARTESIAN_POINT('Ctrl Pts',(-1.0478890117056,0.243040084360927,5.32096628655212));
#8159=CARTESIAN_POINT('Ctrl Pts',(-1.01434736252641,-0.350907601135237,
5.35145773998857));
#8160=CARTESIAN_POINT('Ctrl Pts',(-0.670720080533004,-0.834934758998085,
5.38188128530446));
#8161=CARTESIAN_POINT('Ctrl Pts',(-0.123502010424964,-1.06137898572475,
5.41223662280484));
#8162=CARTESIAN_POINT('Ctrl Pts',(0.458979922580301,-0.962399495397908,
5.44252287745861));
#8163=CARTESIAN_POINT('Ctrl Pts',(0.898423965887827,-0.569251854562554,
5.4727405859251));
#8164=CARTESIAN_POINT('Ctrl Pts',(1.00678249531561,-0.193014045740111,5.49283838071418));
#8165=CARTESIAN_POINT('Ctrl Pts',(1.0068079216488,-0.0041407693603704,5.50287847890709));
#8166=CARTESIAN_POINT('Ctrl Pts',(0.932826886418256,0.00283195947158155,
2.02155536031992));
#8167=CARTESIAN_POINT('Ctrl Pts',(0.932803305353409,0.177998089311277,2.03086681600614));
#8168=CARTESIAN_POINT('Ctrl Pts',(0.832416926289886,0.526449355831317,2.04947889674723));
#8169=CARTESIAN_POINT('Ctrl Pts',(0.425462368210857,0.890529450601189,2.07746218207928));
#8170=CARTESIAN_POINT('Ctrl Pts',(-0.113680331421872,0.982080962129939,
2.10549185328996));
#8171=CARTESIAN_POINT('Ctrl Pts',(-0.619976540307357,0.772544065442153,
2.13357682839298));
#8172=CARTESIAN_POINT('Ctrl Pts',(-0.937793676005252,0.324817811790029,
2.1617153597137));
#8173=CARTESIAN_POINT('Ctrl Pts',(-0.968789729919569,-0.224425204758645,
2.18991046480974));
#8174=CARTESIAN_POINT('Ctrl Pts',(-0.702281633273633,-0.706978147903316,
2.21816297555692));
#8175=CARTESIAN_POINT('Ctrl Pts',(-0.218891386755124,-0.974319694873083,
2.24647466346303));
#8176=CARTESIAN_POINT('Ctrl Pts',(0.333814568943781,-0.943469504346031,
2.27484678113967));
#8177=CARTESIAN_POINT('Ctrl Pts',(0.786375647775339,-0.62254316688173,2.30328080747615));
#8178=CARTESIAN_POINT('Ctrl Pts',(0.999287584601159,-0.109010364379432,
2.33177786821182));
#8179=CARTESIAN_POINT('Ctrl Pts',(0.906153001363644,0.440580406885506,2.36033953197038));
#8180=CARTESIAN_POINT('Ctrl Pts',(0.596008350255508,0.787384121518291,2.3841950831244));
#8181=CARTESIAN_POINT('Ctrl Pts',(0.26519405894642,0.934970553828525,2.40331371530758));
#8182=CARTESIAN_POINT('Ctrl Pts',(-0.00397354741378065,0.973119533744013,
2.41766940006373));
#8183=CARTESIAN_POINT('Ctrl Pts',(-0.273566744652249,0.93502873494253,2.43204204909921));
#8184=CARTESIAN_POINT('Ctrl Pts',(-0.522400248336806,0.823757746325111,
2.4464318017068));
#8185=CARTESIAN_POINT('Ctrl Pts',(-0.730817383368411,0.647684837741542,
2.46083869981358));
#8186=CARTESIAN_POINT('Ctrl Pts',(-0.922289399192392,0.36171191420862,2.47900280186383));
#8187=CARTESIAN_POINT('Ctrl Pts',(-0.990115280771857,0.0270487089396692,
2.49666133821441));
#8188=CARTESIAN_POINT('Ctrl Pts',(-0.93344377138001,-0.29226896767037,2.51381363816868));
#8189=CARTESIAN_POINT('Ctrl Pts',(-0.800338308713536,-0.588160741791901,
2.53098451463937));
#8190=CARTESIAN_POINT('Ctrl Pts',(-0.502644742748064,-0.878987021396976,
2.55248281477416));
#8191=CARTESIAN_POINT('Ctrl Pts',(-0.0748628151458846,-0.999136993401524,
2.57546548511536));
#8192=CARTESIAN_POINT('Ctrl Pts',(0.413375452637366,-0.930246526757298,
2.60136908260148));
#8193=CARTESIAN_POINT('Ctrl Pts',(0.826056853037204,-0.624555315394363,
2.62733007231111));
#8194=CARTESIAN_POINT('Ctrl Pts',(1.0168419590957,-0.0972852674529773,2.65625128192227));
#8195=CARTESIAN_POINT('Ctrl Pts',(0.941995491232734,0.40123528872719,2.68233928665076));
#8196=CARTESIAN_POINT('Ctrl Pts',(0.636429682017026,0.805122864353395,2.70848641485114));
#8197=CARTESIAN_POINT('Ctrl Pts',(0.225807606948362,0.990184376230355,2.7317813313523));
#8198=CARTESIAN_POINT('Ctrl Pts',(-0.27371468395447,0.994843165208457,2.75803796083437));
#8199=CARTESIAN_POINT('Ctrl Pts',(-0.811295562767927,0.710483997877433,
2.78874044098356));
#8200=CARTESIAN_POINT('Ctrl Pts',(-1.09254471947464,-0.00413748468829043,
2.82687585935908));
#8201=CARTESIAN_POINT('Ctrl Pts',(-0.800710019071887,-0.748493642300563,
2.86661399643152));
#8202=CARTESIAN_POINT('Ctrl Pts',(-0.0781674205730973,-1.09716986953638,
2.90648808960406));
#8203=CARTESIAN_POINT('Ctrl Pts',(0.691367439738533,-0.860372850065677,
2.9464982533936));
#8204=CARTESIAN_POINT('Ctrl Pts',(1.09559718621259,-0.160996041341971,2.98664420509449));
#8205=CARTESIAN_POINT('Ctrl Pts',(0.915963771274089,0.629121386204399,3.02692562208008));
#8206=CARTESIAN_POINT('Ctrl Pts',(0.243844124877269,1.08804711068323,3.06734171283987));
#8207=CARTESIAN_POINT('Ctrl Pts',(-0.47240323087623,0.979478908158574,3.10338643967991));
#8208=CARTESIAN_POINT('Ctrl Pts',(-0.910000320002659,0.550829528387608,
3.13501124859862));
#8209=CARTESIAN_POINT('Ctrl Pts',(-1.06536518427627,0.0492471101455223,
3.16217730264769));
#8210=CARTESIAN_POINT('Ctrl Pts',(-0.960838705697807,-0.467598238213527,
3.18940094649933));
#8211=CARTESIAN_POINT('Ctrl Pts',(-0.65934937746825,-0.826164624702505,
3.21365194639263));
#8212=CARTESIAN_POINT('Ctrl Pts',(-0.192619566100375,-1.05658204389069,
3.24098101787109));
#8213=CARTESIAN_POINT('Ctrl Pts',(0.287953883038658,-1.03716173927374,3.26532513654264));
#8214=CARTESIAN_POINT('Ctrl Pts',(0.786515199786917,-0.738387174635933,
3.29581702917111));
#8215=CARTESIAN_POINT('Ctrl Pts',(1.0627682681574,-0.269950457591334,3.32331568948603));
#8216=CARTESIAN_POINT('Ctrl Pts',(1.03222736433692,0.322770007878815,3.35394076194273));
#8217=CARTESIAN_POINT('Ctrl Pts',(0.754172111200573,0.778605651076345,3.38155794876388));
#8218=CARTESIAN_POINT('Ctrl Pts',(0.290513273528267,1.04611740958465,3.40922867610414));
#8219=CARTESIAN_POINT('Ctrl Pts',(-0.335359646284715,1.06336169172191,3.44157258610646));
#8220=CARTESIAN_POINT('Ctrl Pts',(-0.951983941078512,0.644937022856501,
3.4786243719862));
#8221=CARTESIAN_POINT('Ctrl Pts',(-1.10707031340484,-0.0382267088572197,
3.51345595556107));
#8222=CARTESIAN_POINT('Ctrl Pts',(-0.929495283855687,-0.540997199899391,
3.54137565325151));
#8223=CARTESIAN_POINT('Ctrl Pts',(-0.669049818764436,-0.8445166517426,3.56234258200301));
#8224=CARTESIAN_POINT('Ctrl Pts',(-0.314526844233505,-1.03163152300883,
3.58333707155614));
#8225=CARTESIAN_POINT('Ctrl Pts',(0.128448115091551,-1.08197849543191,3.60669360763323));
#8226=CARTESIAN_POINT('Ctrl Pts',(0.60040054697126,-0.923572454548513,3.63242325159083));
#8227=CARTESIAN_POINT('Ctrl Pts',(0.970355718452742,-0.524664964388033,
3.66053639605977));
#8228=CARTESIAN_POINT('Ctrl Pts',(1.07257858888191,-0.123363125148085,3.68194931382862));
#8229=CARTESIAN_POINT('Ctrl Pts',(1.05306973839567,0.15199342992826,3.69662895181969));
#8230=CARTESIAN_POINT('Ctrl Pts',(1.01156739393715,0.346370357112534,3.70720281308074));
#8231=CARTESIAN_POINT('Ctrl Pts',(0.868732331837759,0.666808155110966,3.72571919069949));
#8232=CARTESIAN_POINT('Ctrl Pts',(0.483879628566754,1.01127896449476,3.7522054917375));
#8233=CARTESIAN_POINT('Ctrl Pts',(-0.12857131584191,1.11542778844378,3.78403970128842));
#8234=CARTESIAN_POINT('Ctrl Pts',(-0.703235081453136,0.877515951502692,
3.81592375908098));
#8235=CARTESIAN_POINT('Ctrl Pts',(-1.06387585411653,0.369502985541506,3.84785557289108));
#8236=CARTESIAN_POINT('Ctrl Pts',(-1.09896190148898,-0.253391176953802,
3.87983352293997));
#8237=CARTESIAN_POINT('Ctrl Pts',(-0.796868983409988,-0.800244509653766,
3.91185571127886));
#8238=CARTESIAN_POINT('Ctrl Pts',(-0.249401044438271,-1.10294610857381,
3.94392028721854));
#8239=CARTESIAN_POINT('Ctrl Pts',(0.375981408272009,-1.06793540537711,3.97602532458088));
#8240=CARTESIAN_POINT('Ctrl Pts',(0.887494631104647,-0.705126302172368,
4.00816887101121));
#8241=CARTESIAN_POINT('Ctrl Pts',(1.12783557019956,-0.125133385342958,4.04034894524235));
#8242=CARTESIAN_POINT('Ctrl Pts',(1.02266005657607,0.494501201713791,4.07256351094201));
#8243=CARTESIAN_POINT('Ctrl Pts',(0.603467469596099,0.963639648177038,4.10481055037349));
#8244=CARTESIAN_POINT('Ctrl Pts',(-0.00156042575409069,1.13805630555576,
4.13708792196456));
#8245=CARTESIAN_POINT('Ctrl Pts',(-0.607394163231413,0.963537549874477,
4.16939369795753));
#8246=CARTESIAN_POINT('Ctrl Pts',(-1.01187486453871,0.510748224645048,4.20052792601527));
#8247=CARTESIAN_POINT('Ctrl Pts',(-1.12684783390284,-0.0580425136282725,
4.23048610732755));
#8248=CARTESIAN_POINT('Ctrl Pts',(-0.962363092043994,-0.589239644075659,
4.2592618020737));
#8249=CARTESIAN_POINT('Ctrl Pts',(-0.497901120763859,-1.04513031762221,
4.29285265406363));
#8250=CARTESIAN_POINT('Ctrl Pts',(0.265414780641501,-1.16017299694639,4.33126650928724));
#8251=CARTESIAN_POINT('Ctrl Pts',(0.984906508993433,-0.670147646454155,
4.37450949010921));
#8252=CARTESIAN_POINT('Ctrl Pts',(1.17829785257441,0.178234358754055,4.41777419186001));
#8253=CARTESIAN_POINT('Ctrl Pts',(0.74334096841188,0.932290366300818,4.46105479234514));
#8254=CARTESIAN_POINT('Ctrl Pts',(-0.089749850748141,1.18925176092741,4.50434628274598));
#8255=CARTESIAN_POINT('Ctrl Pts',(-0.785979921194401,0.852637808144917,
4.54283287791217));
#8256=CARTESIAN_POINT('Ctrl Pts',(-1.09678413718196,0.279114855043184,4.57650810802541));
#8257=CARTESIAN_POINT('Ctrl Pts',(-1.09673130021223,-0.278856026110746,
4.60536977372265));
#8258=CARTESIAN_POINT('Ctrl Pts',(-0.829860168431522,-0.769629991342529,
4.63422895110683));
#8259=CARTESIAN_POINT('Ctrl Pts',(-0.360713606530814,-1.07209234198494,
4.66308348222077));
#8260=CARTESIAN_POINT('Ctrl Pts',(0.195822348541668,-1.11420174957979,4.69193058468913));
#8261=CARTESIAN_POINT('Ctrl Pts',(0.630237211031698,-0.917836549559489,
4.71656627824889));
#8262=CARTESIAN_POINT('Ctrl Pts',(0.895633186161231,-0.636491077288054,
4.73698860804468));
#8263=CARTESIAN_POINT('Ctrl Pts',(1.08412177321864,-0.272871489826572,4.75860802443867));
#8264=CARTESIAN_POINT('Ctrl Pts',(1.11394266799808,0.253195431719909,4.78562493558549));
#8265=CARTESIAN_POINT('Ctrl Pts',(0.80797744806265,0.806563226819446,4.81802760839723));
#8266=CARTESIAN_POINT('Ctrl Pts',(0.255057409915322,1.11208766611089,4.85041166201342));
#8267=CARTESIAN_POINT('Ctrl Pts',(-0.375360011406527,1.07664591176693,4.88277443242993));
#8268=CARTESIAN_POINT('Ctrl Pts',(-0.889872436862409,0.711478850433845,
4.91511397615734));
#8269=CARTESIAN_POINT('Ctrl Pts',(-1.13106879693417,0.129004648892796,4.94742804403158));
#8270=CARTESIAN_POINT('Ctrl Pts',(-1.02547541511561,-0.491986465704221,
4.97971454047685));
#8271=CARTESIAN_POINT('Ctrl Pts',(-0.606065844114821,-0.96117968559332,
5.01197132966905));
#8272=CARTESIAN_POINT('Ctrl Pts',(-0.00190792747688937,-1.13514133907331,
5.04419633657574));
#8273=CARTESIAN_POINT('Ctrl Pts',(0.601563511725319,-0.961184874297887,
5.07638748778849));
#8274=CARTESIAN_POINT('Ctrl Pts',(1.01951677311495,-0.493344052857984,5.10854275472083));
#8275=CARTESIAN_POINT('Ctrl Pts',(1.12437206455613,0.124425076160577,5.14066013263499));
#8276=CARTESIAN_POINT('Ctrl Pts',(0.88477473461175,0.702570826283213,5.17273765929341));
#8277=CARTESIAN_POINT('Ctrl Pts',(0.374970578542117,1.06415151415046,5.20477339242679));
#8278=CARTESIAN_POINT('Ctrl Pts',(-0.248216330495147,1.09902333007776,5.23676544866705));
#8279=CARTESIAN_POINT('Ctrl Pts',(-0.79365941366675,0.79742110391797,5.26871194962692));
#8280=CARTESIAN_POINT('Ctrl Pts',(-1.09458936477043,0.252650565010212,5.30061113031637));
#8281=CARTESIAN_POINT('Ctrl Pts',(-1.05961510152497,-0.367758002763614,
5.33246109735404));
#8282=CARTESIAN_POINT('Ctrl Pts',(-0.700502849367933,-0.87369432558995,
5.364260384324));
#8283=CARTESIAN_POINT('Ctrl Pts',(-0.128229042232588,-1.11057117581653,
5.39600672287796));
#8284=CARTESIAN_POINT('Ctrl Pts',(0.4812925884126,-1.00702848710217,5.42769976907791));
#8285=CARTESIAN_POINT('Ctrl Pts',(0.941404086084559,-0.595482393179593,
5.45933506228865));
#8286=CARTESIAN_POINT('Ctrl Pts',(1.05493386550085,-0.201302816156643,5.48039175829747));
#8287=CARTESIAN_POINT('Ctrl Pts',(1.0549604924824,-0.00351081811190388,
5.49090595660125));
#8288=CARTESIAN_POINT('Ctrl Pts',(0.916369847031328,-0.00102349111045756,
2.09404201605622));
#8289=CARTESIAN_POINT('Ctrl Pts',(0.916346688528236,0.171003742848899,2.10318661477118));
#8290=CARTESIAN_POINT('Ctrl Pts',(0.817707835360784,0.512895716711358,2.12145223875872));
#8291=CARTESIAN_POINT('Ctrl Pts',(0.41920029748926,0.869170209238544,2.14884729591622));
#8292=CARTESIAN_POINT('Ctrl Pts',(-0.107422236712015,0.958431037008827,
2.17622676391991));
#8293=CARTESIAN_POINT('Ctrl Pts',(-0.600746857940946,0.754082977371277,
2.20359747278904));
#8294=CARTESIAN_POINT('Ctrl Pts',(-0.909638270891026,0.31865350810529,2.23095959000811));
#8295=CARTESIAN_POINT('Ctrl Pts',(-0.939549502046027,-0.214226424209876,
2.25831630277396));
#8296=CARTESIAN_POINT('Ctrl Pts',(-0.681405678590222,-0.681304517201164,
2.28566947488182));
#8297=CARTESIAN_POINT('Ctrl Pts',(-0.214358534931351,-0.939427406949708,
2.31302155295729));
#8298=CARTESIAN_POINT('Ctrl Pts',(0.318449240362149,-0.909531728351045,
2.34037479460111));
#8299=CARTESIAN_POINT('Ctrl Pts',(0.753742306192684,-0.600663625481568,
2.36773142222178));
#8300=CARTESIAN_POINT('Ctrl Pts',(0.958021262333031,-0.10755669277854,2.39509395663888));
#8301=CARTESIAN_POINT('Ctrl Pts',(0.86863237642743,0.419049362271387,2.4224642099679));
#8302=CARTESIAN_POINT('Ctrl Pts',(0.571920019213654,0.750656867888804,2.44528213440013));
#8303=CARTESIAN_POINT('Ctrl Pts',(0.255980235250472,0.891581369871216,2.46354143837027));
#8304=CARTESIAN_POINT('Ctrl Pts',(-0.000849208062606655,0.927965626989967,
2.47723951301954));
#8305=CARTESIAN_POINT('Ctrl Pts',(-0.25784438103185,0.89163691871115,2.49094127751245));
#8306=CARTESIAN_POINT('Ctrl Pts',(-0.494833212767144,0.785644887369317,
2.50464698245298));
#8307=CARTESIAN_POINT('Ctrl Pts',(-0.693149427962659,0.618083776493324,
2.51835707335789));
#8308=CARTESIAN_POINT('Ctrl Pts',(-0.875173939491225,0.346184871151078,
2.53562686428944));
#8309=CARTESIAN_POINT('Ctrl Pts',(-0.939531665887204,0.0283479115925304,
2.55239869309082));
#8310=CARTESIAN_POINT('Ctrl Pts',(-0.885762312197225,-0.274533729571816,
2.56866880276681));
#8311=CARTESIAN_POINT('Ctrl Pts',(-0.759584016300259,-0.554994827188533,
2.58494500387052));
#8312=CARTESIAN_POINT('Ctrl Pts',(-0.477657541151781,-0.830327440363872,
2.60530275038326));
#8313=CARTESIAN_POINT('Ctrl Pts',(-0.0731616141952735,-0.943861317503134,
2.62703429354313));
#8314=CARTESIAN_POINT('Ctrl Pts',(0.387950369948457,-0.878766091763475,
2.65149944922312));
#8315=CARTESIAN_POINT('Ctrl Pts',(0.777131349534,-0.590316605789316,2.67598803187672));
#8316=CARTESIAN_POINT('Ctrl Pts',(0.956739044025989,-0.0936873461534193,
2.70322901261928));
#8317=CARTESIAN_POINT('Ctrl Pts',(0.8862663494043,0.37526617083507,2.727771384829));
#8318=CARTESIAN_POINT('Ctrl Pts',(0.599098926797975,0.754728897718691,2.75234086323461));
#8319=CARTESIAN_POINT('Ctrl Pts',(0.21368090376234,0.928370361438052,2.77420537437644));
#8320=CARTESIAN_POINT('Ctrl Pts',(-0.254738122925511,0.93271452307593,2.79882743681787));
#8321=CARTESIAN_POINT('Ctrl Pts',(-0.75828727827768,0.666216656617621,2.82758989707073));
#8322=CARTESIAN_POINT('Ctrl Pts',(-1.02123564536619,-0.00240116619232516,
2.86326862539798));
#8323=CARTESIAN_POINT('Ctrl Pts',(-0.748415847817779,-0.697780968165656,
2.90039680552695));
#8324=CARTESIAN_POINT('Ctrl Pts',(-0.07409131528767,-1.02301638245004,2.93760761266815));
#8325=CARTESIAN_POINT('Ctrl Pts',(0.643203902256486,-0.802146148193398,
2.97490493232259));
#8326=CARTESIAN_POINT('Ctrl Pts',(1.01954723631622,-0.150769416767172,3.01229302565354));
#8327=CARTESIAN_POINT('Ctrl Pts',(0.852292508225827,0.584414907128488,3.04977591907635));
#8328=CARTESIAN_POINT('Ctrl Pts',(0.227276839423578,1.0110674650509,3.08735720401155));
#8329=CARTESIAN_POINT('Ctrl Pts',(-0.438319541939116,0.910113738470391,
3.12085411505228));
#8330=CARTESIAN_POINT('Ctrl Pts',(-0.844801512336328,0.511916553688642,
3.15023160268429));
#8331=CARTESIAN_POINT('Ctrl Pts',(-0.989077176791191,0.0460945198815799,
3.17546084042722));
#8332=CARTESIAN_POINT('Ctrl Pts',(-0.892014438447379,-0.433794636537154,
3.2007381352498));
#8333=CARTESIAN_POINT('Ctrl Pts',(-0.612118438007755,-0.766673921756164,
3.22325206561452));
#8334=CARTESIAN_POINT('Ctrl Pts',(-0.178857765623275,-0.980565792531451,
3.24862139375817));
#8335=CARTESIAN_POINT('Ctrl Pts',(0.267228106207802,-0.962539184921591,
3.27121838614417));
#8336=CARTESIAN_POINT('Ctrl Pts',(0.730013939585809,-0.685206821667964,
3.29952225272199));
#8337=CARTESIAN_POINT('Ctrl Pts',(0.986464765139846,-0.250369071743527,
3.32504870915495));
#8338=CARTESIAN_POINT('Ctrl Pts',(0.95812182499081,0.299918184836265,3.35348122127316));
#8339=CARTESIAN_POINT('Ctrl Pts',(0.69994234794655,0.723197169461558,3.37912524154526));
#8340=CARTESIAN_POINT('Ctrl Pts',(0.26932018482604,0.971666495969792,3.40482455316389));
#8341=CARTESIAN_POINT('Ctrl Pts',(-0.31212188900552,0.98771052697221,3.43487218195244));
#8342=CARTESIAN_POINT('Ctrl Pts',(-0.885238845826609,0.598894963282439,
3.46930673479697));
#8343=CARTESIAN_POINT('Ctrl Pts',(-1.02953961553121,-0.0363787851602884,
3.5016965523722));
#8344=CARTESIAN_POINT('Ctrl Pts',(-0.864336764959382,-0.504181293959062,
3.52767346931298));
#8345=CARTESIAN_POINT('Ctrl Pts',(-0.621930095431672,-0.786700433736122,
3.54718892278537));
#8346=CARTESIAN_POINT('Ctrl Pts',(-0.291824674843086,-0.960947772200679,
3.56673743356965));
#8347=CARTESIAN_POINT('Ctrl Pts',(0.120824733563513,-1.00786799696591,3.58849479474554));
#8348=CARTESIAN_POINT('Ctrl Pts',(0.560718250558898,-0.860264176152269,
3.61247534427901));
#8349=CARTESIAN_POINT('Ctrl Pts',(0.90579561929086,-0.488243207438898,3.63869541996055));
#8350=CARTESIAN_POINT('Ctrl Pts',(1.00123268399749,-0.113720390961006,3.65867897605182));
#8351=CARTESIAN_POINT('Ctrl Pts',(0.983017585188276,0.143402603591866,3.67238638521822));
#8352=CARTESIAN_POINT('Ctrl Pts',(0.944256590238532,0.324946829770906,3.68226204628741));
#8353=CARTESIAN_POINT('Ctrl Pts',(0.810820991239849,0.624325964678426,3.69956105418397));
#8354=CARTESIAN_POINT('Ctrl Pts',(0.451074214704145,0.946410697051131,3.72432137261343));
#8355=CARTESIAN_POINT('Ctrl Pts',(-0.12202991938042,1.04395262161911,3.75411010316036));
#8356=CARTESIAN_POINT('Ctrl Pts',(-0.660359762621321,0.821174393840838,
3.78397519806004));
#8357=CARTESIAN_POINT('Ctrl Pts',(-0.998609248217651,0.344859144986669,
3.8139167304214));
#8358=CARTESIAN_POINT('Ctrl Pts',(-1.03164097244784,-0.239875733016347,
3.84393465319117));
#8359=CARTESIAN_POINT('Ctrl Pts',(-0.747811121324658,-0.753874860605696,
3.8740288769748));
#8360=CARTESIAN_POINT('Ctrl Pts',(-0.232712138351297,-1.03879805778991,
3.90419923342449));
#8361=CARTESIAN_POINT('Ctrl Pts',(0.356495892757353,-1.00592070547447,3.9344454910798));
#8362=CARTESIAN_POINT('Ctrl Pts',(0.839107848540948,-0.663748333283532,
3.96476735078991));
#8363=CARTESIAN_POINT('Ctrl Pts',(1.06625077284666,-0.115907777840236,3.99516444147537));
#8364=CARTESIAN_POINT('Ctrl Pts',(0.966878330006049,0.470257402286813,4.02563633586024));
#8365=CARTESIAN_POINT('Ctrl Pts',(0.569866293499877,0.914758605400251,4.05618251087602));
#8366=CARTESIAN_POINT('Ctrl Pts',(-0.00408784481252405,1.08035069145649,
4.08680243863468));
#8367=CARTESIAN_POINT('Ctrl Pts',(-0.579750345963528,0.914663327800101,
4.11749538541984));
#8368=CARTESIAN_POINT('Ctrl Pts',(-0.964749041164902,0.483870415823376,
4.14712137732599));
#8369=CARTESIAN_POINT('Ctrl Pts',(-1.0744299924881,-0.0581826966804888,
4.17567030962805));
#8370=CARTESIAN_POINT('Ctrl Pts',(-0.917518259249771,-0.565200962277581,
4.2031340732151));
#8371=CARTESIAN_POINT('Ctrl Pts',(-0.473682144476704,-1.00103453406579,
4.23523938847692));
#8372=CARTESIAN_POINT('Ctrl Pts',(0.257222988296793,-1.11148785556699,4.27202226579617));
#8373=CARTESIAN_POINT('Ctrl Pts',(0.947986891210012,-0.641485758789489,
4.31352348095811));
#8374=CARTESIAN_POINT('Ctrl Pts',(1.13439835811232,0.174626964839297,4.35514289607299));
#8375=CARTESIAN_POINT('Ctrl Pts',(0.715278455463992,0.901996673495511,4.3968779276954));
#8376=CARTESIAN_POINT('Ctrl Pts',(-0.0899753508703297,1.15079804708479,
4.43872545034349));
#8377=CARTESIAN_POINT('Ctrl Pts',(-0.764860835418986,0.824889245468528,
4.47602022241449));
#8378=CARTESIAN_POINT('Ctrl Pts',(-1.06684896287779,0.26796150264565,4.50872224677515));
#8379=CARTESIAN_POINT('Ctrl Pts',(-1.0669019032667,-0.274863137816934,4.5367995180593));
#8380=CARTESIAN_POINT('Ctrl Pts',(-0.806952932018616,-0.75318333934492,
4.56492138454683));
#8381=CARTESIAN_POINT('Ctrl Pts',(-0.349034088477564,-1.04854060213485,
4.59308718022527));
#8382=CARTESIAN_POINT('Ctrl Pts',(0.195199242947889,-1.08984580813762,4.62129657098129));
#8383=CARTESIAN_POINT('Ctrl Pts',(0.620780261672434,-0.897578145268399,
4.64542615597834));
#8384=CARTESIAN_POINT('Ctrl Pts',(0.881157012154678,-0.621593420716843,
4.66545991481029));
#8385=CARTESIAN_POINT('Ctrl Pts',(1.06627072006747,-0.264543937473019,4.68668883949075));
#8386=CARTESIAN_POINT('Ctrl Pts',(1.09573971133967,0.252780133526497,4.71325480051859));
#8387=CARTESIAN_POINT('Ctrl Pts',(0.794394693978023,0.798163977577909,4.74518261070608));
#8388=CARTESIAN_POINT('Ctrl Pts',(0.248519420266219,1.09999436085071,4.77715633733294));
#8389=CARTESIAN_POINT('Ctrl Pts',(-0.375240449586358,1.06510654881083,4.80917449611883));
#8390=CARTESIAN_POINT('Ctrl Pts',(-0.885457074079279,0.703208795097844,
4.84123501597506));
#8391=CARTESIAN_POINT('Ctrl Pts',(-1.12524810993215,0.124601555468318,4.87333605018736));
#8392=CARTESIAN_POINT('Ctrl Pts',(-1.02030690402006,-0.493639120147483,
4.90547560083362));
#8393=CARTESIAN_POINT('Ctrl Pts',(-0.602052162605231,-0.961813726065453,
4.93765169075804));
#8394=CARTESIAN_POINT('Ctrl Pts',(0.00182870667745636,-1.135885393394,4.9698622965679));
#8395=CARTESIAN_POINT('Ctrl Pts',(0.606367058350047,-0.961811168634456,
5.00210536221374));
#8396=CARTESIAN_POINT('Ctrl Pts',(1.02602213787626,-0.492338924724964,5.03437880857729));
#8397=CARTESIAN_POINT('Ctrl Pts',(1.13166612893175,0.128989441018504,5.06668052554289));
#8398=CARTESIAN_POINT('Ctrl Pts',(0.89034970584236,0.711757684128376,5.09900838789433));
#8399=CARTESIAN_POINT('Ctrl Pts',(0.375583834764511,1.07707957256597,5.13136022647449));
#8400=CARTESIAN_POINT('Ctrl Pts',(-0.255070373989398,1.1125503833894,5.16373388639704));
#8401=CARTESIAN_POINT('Ctrl Pts',(-0.808266612488616,0.806867014603004,
5.19612713158992));
#8402=CARTESIAN_POINT('Ctrl Pts',(-1.11420070816338,0.253411220794365,5.22853784854267));
#8403=CARTESIAN_POINT('Ctrl Pts',(-1.07877100089406,-0.378265696239001,
5.26096359350033));
#8404=CARTESIAN_POINT('Ctrl Pts',(-0.712560292595334,-0.894509866678123,
5.29340262757595));
#8405=CARTESIAN_POINT('Ctrl Pts',(-0.127650607355885,-1.13681080552691,
5.32585163203065));
#8406=CARTESIAN_POINT('Ctrl Pts',(0.496644911088633,-1.03091288864219,5.35831080085294));
#8407=CARTESIAN_POINT('Ctrl Pts',(0.968925991004248,-0.608726803401192,
5.39077254625792));
#8408=CARTESIAN_POINT('Ctrl Pts',(1.08573126301311,-0.203385678647448,5.41242485487802));
#8409=CARTESIAN_POINT('Ctrl Pts',(1.08575865405747,8.19725653867553E-5,
5.42324075872855));
#8410=CARTESIAN_POINT('Ctrl Pts',(0.962721347542879,-0.00411661163177441,
2.15234685977571));
#8411=CARTESIAN_POINT('Ctrl Pts',(0.962697036439002,0.17647243326112,2.16194658599263));
#8412=CARTESIAN_POINT('Ctrl Pts',(0.859106513837746,0.53539067596772,2.18112130305809));
#8413=CARTESIAN_POINT('Ctrl Pts',(0.441523188737198,0.908498155871786,2.20981828668204));
#8414=CARTESIAN_POINT('Ctrl Pts',(-0.109164096041492,1.00171508855228,2.23844766404908));
#8415=CARTESIAN_POINT('Ctrl Pts',(-0.623968541999703,0.788299051013983,
2.26701152025929));
#8416=CARTESIAN_POINT('Ctrl Pts',(-0.945582885707644,0.334666298512384,
2.29551065902089));
#8417=CARTESIAN_POINT('Ctrl Pts',(-0.976516553994219,-0.219280947897082,
2.3239465404964));
#8418=CARTESIAN_POINT('Ctrl Pts',(-0.708579872107489,-0.70374057431398,
2.35232039322412));
#8419=CARTESIAN_POINT('Ctrl Pts',(-0.225007223597382,-0.970809187175863,
2.3806336417432));
#8420=CARTESIAN_POINT('Ctrl Pts',(0.325378852667097,-0.93976097174502,2.40888765462467));
#8421=CARTESIAN_POINT('Ctrl Pts',(0.773967917830734,-0.621252530146527,
2.43708398784343));
#8422=CARTESIAN_POINT('Ctrl Pts',(0.983916611731044,-0.114028404154294,
2.46522395532223));
#8423=CARTESIAN_POINT('Ctrl Pts',(0.892012622004092,0.426349139204185,2.49330953081928));
#8424=CARTESIAN_POINT('Ctrl Pts',(0.588120879377049,0.765771851692147,2.51666932886635));
#8425=CARTESIAN_POINT('Ctrl Pts',(0.265171410425461,0.909790782859939,2.53533257394823));
#8426=CARTESIAN_POINT('Ctrl Pts',(0.00295104918847766,0.946918837023357,
2.54931723993354));
#8427=CARTESIAN_POINT('Ctrl Pts',(-0.259128227762097,0.909851006157386,
2.56328950518113));
#8428=CARTESIAN_POINT('Ctrl Pts',(-0.500519402075947,0.801866490451361,
2.57724962652205));
#8429=CARTESIAN_POINT('Ctrl Pts',(-0.702277143832267,0.631373250483782,
2.5911976605843));
#8430=CARTESIAN_POINT('Ctrl Pts',(-0.88723717920968,0.355036238046743,2.60874752373027));
#8431=CARTESIAN_POINT('Ctrl Pts',(-0.952446153747716,0.0325776524498273,
2.62575995705517));
#8432=CARTESIAN_POINT('Ctrl Pts',(-0.897957539757315,-0.274233551693925,
2.64224109774197));
#8433=CARTESIAN_POINT('Ctrl Pts',(-0.770255823431421,-0.558036376433486,
2.65871051814366));
#8434=CARTESIAN_POINT('Ctrl Pts',(-0.485357076941816,-0.836110903690922,
2.67927513518536));
#8435=CARTESIAN_POINT('Ctrl Pts',(-0.0775319663989175,-0.950476259880596,
2.7011828579738));
#8436=CARTESIAN_POINT('Ctrl Pts',(0.386529697138345,-0.884891476815102,
2.7258038844267));
#8437=CARTESIAN_POINT('Ctrl Pts',(0.777236927466001,-0.595055584395186,
2.75039346878802));
#8438=CARTESIAN_POINT('Ctrl Pts',(0.956995355922048,-0.097529407098393,
2.77767868535629));
#8439=CARTESIAN_POINT('Ctrl Pts',(0.886438324246732,0.371210169594461,2.80220878560151));
#8440=CARTESIAN_POINT('Ctrl Pts',(0.599889044325121,0.749619302024166,2.8267136473443));
#8441=CARTESIAN_POINT('Ctrl Pts',(0.216229858198713,0.92235427561694,2.84847500153269));
#8442=CARTESIAN_POINT('Ctrl Pts',(-0.249196296007761,0.926605057610193,
2.87293857301302));
#8443=CARTESIAN_POINT('Ctrl Pts',(-0.748339976156685,0.662149208528223,
2.90145349416336));
#8444=CARTESIAN_POINT('Ctrl Pts',(-1.00784252719217,0.00108226136453731,
2.93671648399365));
#8445=CARTESIAN_POINT('Ctrl Pts',(-0.738609749853676,-0.683953218299274,
2.97329856217955));
#8446=CARTESIAN_POINT('Ctrl Pts',(-0.0760369512723759,-1.0030387720919,
3.00984720605691));
#8447=CARTESIAN_POINT('Ctrl Pts',(0.626253849277891,-0.78633880600751,3.04636816423152));
#8448=CARTESIAN_POINT('Ctrl Pts',(0.993305041368912,-0.150207345540429,
3.08286657411111));
#8449=CARTESIAN_POINT('Ctrl Pts',(0.830107070720763,0.565297577569166,3.1193475619553));
#8450=CARTESIAN_POINT('Ctrl Pts',(0.223310847090626,0.979012770835039,3.15581708462796));
#8451=CARTESIAN_POINT('Ctrl Pts',(-0.420703939193676,0.880994726407311,
3.18822751837814));
#8452=CARTESIAN_POINT('Ctrl Pts',(-0.813020823197554,0.496480837443196,
3.21658791513038));
#8453=CARTESIAN_POINT('Ctrl Pts',(-0.95195527204512,0.0475836205868763,
3.24089647232581));
#8454=CARTESIAN_POINT('Ctrl Pts',(-0.858475820711094,-0.413990349512743,
3.26521013485892));
#8455=CARTESIAN_POINT('Ctrl Pts',(-0.58969183309083,-0.733533759079077,
3.28682351737405));
#8456=CARTESIAN_POINT('Ctrl Pts',(-0.174261433996607,-0.938557040943953,
3.31114684834291));
#8457=CARTESIAN_POINT('Ctrl Pts',(0.252658678818904,-0.92116569916459,3.33277106740655));
#8458=CARTESIAN_POINT('Ctrl Pts',(0.694802991231644,-0.656123967968513,
3.35981348087761));
#8459=CARTESIAN_POINT('Ctrl Pts',(0.939291519468958,-0.241256077865081,
3.38416158448978));
#8460=CARTESIAN_POINT('Ctrl Pts',(0.91218681845093,0.282668180662149,3.41123151679007));
#8461=CARTESIAN_POINT('Ctrl Pts',(0.666683572839207,0.68499526322474,3.43560763134909));
#8462=CARTESIAN_POINT('Ctrl Pts',(0.257903664472838,0.920757528699098,3.45999919062152));
#8463=CARTESIAN_POINT('Ctrl Pts',(-0.293190683850414,0.935856697443789,
3.48847629875965));
#8464=CARTESIAN_POINT('Ctrl Pts',(-0.835253605337006,0.567793133594608,
3.52105113144131));
#8465=CARTESIAN_POINT('Ctrl Pts',(-0.971269459465228,-0.0320272028560387,
3.5516285035243));
#8466=CARTESIAN_POINT('Ctrl Pts',(-0.815479303068769,-0.473036420310123,
3.57611817473918));
#8467=CARTESIAN_POINT('Ctrl Pts',(-0.587134159411761,-0.73912653502778,
3.59449938665691));
#8468=CARTESIAN_POINT('Ctrl Pts',(-0.276488049756515,-0.903067474146875,
3.61289387563012));
#8469=CARTESIAN_POINT('Ctrl Pts',(0.111480528612638,-0.94714988836231,3.63334893620245));
#8470=CARTESIAN_POINT('Ctrl Pts',(0.524623823248839,-0.808457946093702,
3.65587122236952));
#8471=CARTESIAN_POINT('Ctrl Pts',(0.848331491884379,-0.459374496378889,
3.68047110361084));
#8472=CARTESIAN_POINT('Ctrl Pts',(0.937726582189932,-0.108362961515514,
3.699198284524));
#8473=CARTESIAN_POINT('Ctrl Pts',(0.920661842541678,0.132470309013187,3.71203717388858));
#8474=CARTESIAN_POINT('Ctrl Pts',(0.884364839801641,0.30246672743071,3.7212845535523));
#8475=CARTESIAN_POINT('Ctrl Pts',(0.759456347652235,0.582682043325935,3.73747601951444));
#8476=CARTESIAN_POINT('Ctrl Pts',(0.422964808729093,0.883858075393611,3.76063152662413));
#8477=CARTESIAN_POINT('Ctrl Pts',(-0.112512540933623,0.974918894479097,
3.78846289755193));
#8478=CARTESIAN_POINT('Ctrl Pts',(-0.614996115744401,0.766897370709679,
3.81633979986252));
#8479=CARTESIAN_POINT('Ctrl Pts',(-0.930417714207424,0.322614824716656,
3.84426444412183));
#8480=CARTESIAN_POINT('Ctrl Pts',(-0.961140988257394,-0.222324918431914,
3.87223838421193));
#8481=CARTESIAN_POINT('Ctrl Pts',(-0.69677120594697,-0.700969958174984,
3.9002634148559));
#8482=CARTESIAN_POINT('Ctrl Pts',(-0.217362760794632,-0.96609476978467,
3.92834117714213));
#8483=CARTESIAN_POINT('Ctrl Pts',(0.330671812874561,-0.935470664097115,
3.95647331440789));
#8484=CARTESIAN_POINT('Ctrl Pts',(0.779309073310336,-0.617338693461153,
3.98466140544244));
#8485=CARTESIAN_POINT('Ctrl Pts',(0.990347687928942,-0.108251830746577,
4.01290698107989));
#8486=CARTESIAN_POINT('Ctrl Pts',(0.898013637895048,0.436226331588933,4.04121153220018));
#8487=CARTESIAN_POINT('Ctrl Pts',(0.529328619401076,0.84897754575353,4.06957647148122));
#8488=CARTESIAN_POINT('Ctrl Pts',(-0.00352717617365774,1.00269376187457,
4.09800320508173));
#8489=CARTESIAN_POINT('Ctrl Pts',(-0.53787017868102,0.848886205494921,4.12649296047967));
#8490=CARTESIAN_POINT('Ctrl Pts',(-0.895195474546552,0.44904748125299,4.15398961563631));
#8491=CARTESIAN_POINT('Ctrl Pts',(-0.99698925472466,-0.0540344302060386,
4.18048581348479));
#8492=CARTESIAN_POINT('Ctrl Pts',(-0.851356000818643,-0.524614091200913,
4.20597562966137));
#8493=CARTESIAN_POINT('Ctrl Pts',(-0.439393797688116,-0.929156781447132,
4.23577571608365));
#8494=CARTESIAN_POINT('Ctrl Pts',(0.239134479307232,-1.03172425268404,4.26992283604039));
#8495=CARTESIAN_POINT('Ctrl Pts',(0.88062635002243,-0.595308924912992,4.30846235818722));
#8496=CARTESIAN_POINT('Ctrl Pts',(1.05387305271645,0.162865133152882,4.34712801875718));
#8497=CARTESIAN_POINT('Ctrl Pts',(0.664364503263854,0.839011374927392,4.38592206739164));
#8498=CARTESIAN_POINT('Ctrl Pts',(-0.0845907046652596,1.07052624790495,
4.42484600837287));
#8499=CARTESIAN_POINT('Ctrl Pts',(-0.712842695379716,0.767247970283082,
4.45956176146268));
#8500=CARTESIAN_POINT('Ctrl Pts',(-0.994185348275163,0.248487058242295,
4.49002428484184));
#8501=CARTESIAN_POINT('Ctrl Pts',(-0.994274270717777,-0.257467969569223,
4.51619461558179));
#8502=CARTESIAN_POINT('Ctrl Pts',(-0.751855150970942,-0.70361733908245,
4.54242443744114));
#8503=CARTESIAN_POINT('Ctrl Pts',(-0.324470129231318,-0.979336141683844,
4.56871404297466));
#8504=CARTESIAN_POINT('Ctrl Pts',(0.183878891843407,-1.0179645870293,4.59506396293236));
#8505=CARTESIAN_POINT('Ctrl Pts',(0.581751730736977,-0.838265598761856,
4.61762222395677));
#8506=CARTESIAN_POINT('Ctrl Pts',(0.825328076283757,-0.580104449599382,
4.63636280804653));
#8507=CARTESIAN_POINT('Ctrl Pts',(0.998586089801493,-0.245951087937804,
4.65623122227954));
#8508=CARTESIAN_POINT('Ctrl Pts',(1.02625485131006,0.238581037359652,4.68111440254546));
#8509=CARTESIAN_POINT('Ctrl Pts',(0.743789931407803,0.74997765265919,4.7110508969794));
#8510=CARTESIAN_POINT('Ctrl Pts',(0.231451184999164,1.03337076367631,4.74106392441336));
#8511=CARTESIAN_POINT('Ctrl Pts',(-0.354721818349007,1.0006818484025,4.7711534400235));
#8512=CARTESIAN_POINT('Ctrl Pts',(-0.834827143804072,0.660265838075267,
4.80131925998906));
#8513=CARTESIAN_POINT('Ctrl Pts',(-1.06081927769198,0.115228410684275,4.83156116578106));
#8514=CARTESIAN_POINT('Ctrl Pts',(-0.961937848645582,-0.467962848556256,
4.86187885676498));
#8515=CARTESIAN_POINT('Ctrl Pts',(-0.566959468281633,-0.910252364800106,
4.89227197078685));
#8516=CARTESIAN_POINT('Ctrl Pts',(0.00419774968818196,-1.07501280772215,
4.92274007833275));
#8517=CARTESIAN_POINT('Ctrl Pts',(0.576862797925814,-0.910241916881616,
4.95328268065342));
#8518=CARTESIAN_POINT('Ctrl Pts',(0.975048407214078,-0.464974479905994,
4.98389921569725));
#8519=CARTESIAN_POINT('Ctrl Pts',(1.07554249229,0.125301228542384,5.01458905199364));
#8520=CARTESIAN_POINT('Ctrl Pts',(0.846043667387722,0.679874836165035,5.04535150127358));
#8521=CARTESIAN_POINT('Ctrl Pts',(0.355525902562435,1.02815400916832,5.07618579327906));
#8522=CARTESIAN_POINT('Ctrl Pts',(-0.246487037256726,1.06215264226365,5.10709113070068));
#8523=CARTESIAN_POINT('Ctrl Pts',(-0.775512215175448,0.769987306507226,
5.13806658010937));
#8524=CARTESIAN_POINT('Ctrl Pts',(-1.06866263704341,0.239955456649329,5.16911131550179));
#8525=CARTESIAN_POINT('Ctrl Pts',(-1.03481521163521,-0.366119450751765,
5.20022407990668));
#8526=CARTESIAN_POINT('Ctrl Pts',(-0.682953505990723,-0.862389869623227,
5.23140440347673));
#8527=CARTESIAN_POINT('Ctrl Pts',(-0.119822206743421,-1.09583181987539,
5.26264991422472));
#8528=CARTESIAN_POINT('Ctrl Pts',(0.482414728890113,-0.99383199184833,5.29396235184144));
#8529=CARTESIAN_POINT('Ctrl Pts',(0.938933400305489,-0.585955811533194,
5.32533420344708));
#8530=CARTESIAN_POINT('Ctrl Pts',(1.05214732608714,-0.193544083814575,5.34629921120176));
#8531=CARTESIAN_POINT('Ctrl Pts',(1.05217386845809,0.00361940518297847,
5.35677999931289));
#8532=CARTESIAN_POINT('Ctrl Pts',(1.03720012607221,-0.00409632044393359,
2.15215376000718));
#8533=CARTESIAN_POINT('Ctrl Pts',(1.0371739562621,0.190299665690889,2.1624874336011));
#8534=CARTESIAN_POINT('Ctrl Pts',(0.92558272158616,0.577069833109404,2.18315020057125));
#8535=CARTESIAN_POINT('Ctrl Pts',(0.475702554611024,0.978996718760897,2.21406476939329));
#8536=CARTESIAN_POINT('Ctrl Pts',(-0.117602071922459,1.0794537551305,2.24491151338212));
#8537=CARTESIAN_POINT('Ctrl Pts',(-0.67223251082179,0.849511405004554,2.27568514165904));
#8538=CARTESIAN_POINT('Ctrl Pts',(-1.01868605409155,0.360824868161801,2.30638700631186));
#8539=CARTESIAN_POINT('Ctrl Pts',(-1.05198527374106,-0.235832800197401,
2.33701552683969));
#8540=CARTESIAN_POINT('Ctrl Pts',(-0.763435051280867,-0.757511025548864,
2.36757050042531));
#8541=CARTESIAN_POINT('Ctrl Pts',(-0.242837916088414,-1.0449929062352,2.39805118245125));
#8542=CARTESIAN_POINT('Ctrl Pts',(0.349453096149757,-1.01154391433838,2.42845715295811));
#8543=CARTESIAN_POINT('Ctrl Pts',(0.83196489491292,-0.668897917475794,2.45878794166022));
#8544=CARTESIAN_POINT('Ctrl Pts',(1.05764301678683,-0.123543606707892,2.48904318489043));
#8545=CARTESIAN_POINT('Ctrl Pts',(0.958836971515402,0.457095916413721,2.51922258240279));
#8546=CARTESIAN_POINT('Ctrl Pts',(0.632465576049352,0.821551271589622,2.54430864803126));
#8547=CARTESIAN_POINT('Ctrl Pts',(0.285855566773319,0.976108708850338,2.56433940263466));
#8548=CARTESIAN_POINT('Ctrl Pts',(0.00452756006785972,1.01593379748638,
2.57934338276949));
#8549=CARTESIAN_POINT('Ctrl Pts',(-0.2765370042666,0.976170788344264,2.59432827452502));
#8550=CARTESIAN_POINT('Ctrl Pts',(-0.535307761035302,0.86040144442448,2.60929405779257));
#8551=CARTESIAN_POINT('Ctrl Pts',(-0.751497261576938,0.677699097345559,
2.62424075774338));
#8552=CARTESIAN_POINT('Ctrl Pts',(-0.949595343425886,0.381711610440999,
2.64303841886695));
#8553=CARTESIAN_POINT('Ctrl Pts',(-1.01936200319434,0.0365227623030728,
2.66125102072396));
#8554=CARTESIAN_POINT('Ctrl Pts',(-0.961064851420158,-0.291671978015799,
2.67888133848244));
#8555=CARTESIAN_POINT('Ctrl Pts',(-0.824511437821258,-0.595122439806544,
2.6964916259616));
#8556=CARTESIAN_POINT('Ctrl Pts',(-0.520048507305593,-0.892224089661673,
2.71846705734819));
#8557=CARTESIAN_POINT('Ctrl Pts',(-0.0846891312651837,-1.01424813098015,
2.74185404671718));
#8558=CARTESIAN_POINT('Ctrl Pts',(0.410258207256074,-0.944271157163008,
2.76811431360273));
#8559=CARTESIAN_POINT('Ctrl Pts',(0.826474742453967,-0.635355915055917,
2.79431536270512));
#8560=CARTESIAN_POINT('Ctrl Pts',(1.0176655081718,-0.105925126889566,2.82335070844217));
#8561=CARTESIAN_POINT('Ctrl Pts',(0.942602044217525,0.392253570097308,2.8494235300747));
#8562=CARTESIAN_POINT('Ctrl Pts',(0.638357555434203,0.793903498901933,2.87543765808239));
#8563=CARTESIAN_POINT('Ctrl Pts',(0.231584750247889,0.976964213416025,2.89850945113229));
#8564=CARTESIAN_POINT('Ctrl Pts',(-0.261300417458962,0.981432732038026,
2.92441673147305));
#8565=CARTESIAN_POINT('Ctrl Pts',(-0.78911757047424,0.701577318097918,2.95457534274698));
#8566=CARTESIAN_POINT('Ctrl Pts',(-1.06274273585526,0.00369915306037486,
2.99179914126635));
#8567=CARTESIAN_POINT('Ctrl Pts',(-0.778888284969809,-0.717626824525481,
3.03032832205921));
#8568=CARTESIAN_POINT('Ctrl Pts',(-0.0825571702149149,-1.05259129336624,
3.06873400475036));
#8569=CARTESIAN_POINT('Ctrl Pts',(0.653482636017743,-0.82510163125457,3.10701834952163));
#8570=CARTESIAN_POINT('Ctrl Pts',(1.03694987840345,-0.159780933193991,3.14518392884017));
#8571=CARTESIAN_POINT('Ctrl Pts',(0.866376317169457,0.586342300918658,3.1832336854523));
#8572=CARTESIAN_POINT('Ctrl Pts',(0.234998019991916,1.01633566146955,3.22117007239323));
#8573=CARTESIAN_POINT('Ctrl Pts',(-0.432991952034301,0.914309265779491,
3.25479444760821));
#8574=CARTESIAN_POINT('Ctrl Pts',(-0.838878119080994,0.516296390053429,
3.2841451151001));
#8575=CARTESIAN_POINT('Ctrl Pts',(-0.982273687442794,0.0525680030763169,
3.30925761409405));
#8576=CARTESIAN_POINT('Ctrl Pts',(-0.885793450990451,-0.423240964042453,
3.33432279750852));
#8577=CARTESIAN_POINT('Ctrl Pts',(-0.609137316783548,-0.751973908577496,
3.35656577614145));
#8578=CARTESIAN_POINT('Ctrl Pts',(-0.182387946913773,-0.962521184839306,
3.38155029819673));
#8579=CARTESIAN_POINT('Ctrl Pts',(0.255309527200463,-0.944507833568579,
3.40372342590835));
#8580=CARTESIAN_POINT('Ctrl Pts',(0.707637937756388,-0.673273572524831,
3.43139261558955));
#8581=CARTESIAN_POINT('Ctrl Pts',(0.95709097082737,-0.249569786756698,3.45625502960754));
#8582=CARTESIAN_POINT('Ctrl Pts',(0.929340031620981,0.2840721590868,3.48382950356397));
#8583=CARTESIAN_POINT('Ctrl Pts',(0.679684036454164,0.692970704905364,3.50860996446133));
#8584=CARTESIAN_POINT('Ctrl Pts',(0.264972950420313,0.932018810712846,3.53335442277599));
#8585=CARTESIAN_POINT('Ctrl Pts',(-0.292875541075979,0.947146888293306,
3.56218205848296));
#8586=CARTESIAN_POINT('Ctrl Pts',(-0.83992957344522,0.575232532689319,3.59507362871049));
#8587=CARTESIAN_POINT('Ctrl Pts',(-0.976446149645535,-0.0285021060551591,
3.62585138286231));
#8588=CARTESIAN_POINT('Ctrl Pts',(-0.819982137782929,-0.471194465906437,
3.65043867935641));
#8589=CARTESIAN_POINT('Ctrl Pts',(-0.591068510913671,-0.737865206766389,
3.66886289728087));
#8590=CARTESIAN_POINT('Ctrl Pts',(-0.28016561471819,-0.901875466186263,
3.68727288345947));
#8591=CARTESIAN_POINT('Ctrl Pts',(0.107481257946226,-0.945857362484449,
3.70771184020532));
#8592=CARTESIAN_POINT('Ctrl Pts',(0.519462496772379,-0.807428539347808,
3.73017500517365));
#8593=CARTESIAN_POINT('Ctrl Pts',(0.841496073287022,-0.459974006299116,
3.75465525952053));
#8594=CARTESIAN_POINT('Ctrl Pts',(0.93019017290814,-0.111360958781802,3.77325611214999));
#8595=CARTESIAN_POINT('Ctrl Pts',(0.913264927019297,0.127451186282573,3.78598775165775));
#8596=CARTESIAN_POINT('Ctrl Pts',(0.877290869596397,0.295921312263089,3.79515241068551));
#8597=CARTESIAN_POINT('Ctrl Pts',(0.753583159450096,0.573375486738159,3.8111856372686));
#8598=CARTESIAN_POINT('Ctrl Pts',(0.420870761936589,0.870973318960077,3.83407713920392));
#8599=CARTESIAN_POINT('Ctrl Pts',(-0.10719372434703,0.960591213795104,3.86152417393542));
#8600=CARTESIAN_POINT('Ctrl Pts',(-0.601464341491623,0.755785630251061,
3.88895202302946));
#8601=CARTESIAN_POINT('Ctrl Pts',(-0.910906330100926,0.319626006652346,
3.91636240063127));
#8602=CARTESIAN_POINT('Ctrl Pts',(-0.940819883683162,-0.214000382719056,
3.94375782125121));
#8603=CARTESIAN_POINT('Ctrl Pts',(-0.682385307441754,-0.681546976981073,
3.97114042705916));
#8604=CARTESIAN_POINT('Ctrl Pts',(-0.214987241307903,-0.939836825243413,
3.99851254259768));
#8605=CARTESIAN_POINT('Ctrl Pts',(0.318023095443073,-0.909885582634909,
4.02587641384691));
#8606=CARTESIAN_POINT('Ctrl Pts',(0.7533132090918,-0.601017068726198,4.05323432668543));
#8607=CARTESIAN_POINT('Ctrl Pts',(0.957524926712381,-0.10797780366471,4.0805885629404));
#8608=CARTESIAN_POINT('Ctrl Pts',(0.868146657813169,0.418119687888217,4.1079413947471));
#8609=CARTESIAN_POINT('Ctrl Pts',(0.51252087301969,0.816016703834251,4.13529515584408));
#8610=CARTESIAN_POINT('Ctrl Pts',(-0.000280531296823317,0.96378804214646,
4.16265203940924));
#8611=CARTESIAN_POINT('Ctrl Pts',(-0.513389900953546,0.815932837409874,
4.19001455783718));
#8612=CARTESIAN_POINT('Ctrl Pts',(-0.855769768104171,0.432614499437845,
4.21637087266359));
#8613=CARTESIAN_POINT('Ctrl Pts',(-0.953045996844169,-0.0487133751138879,
4.2417227597978));
#8614=CARTESIAN_POINT('Ctrl Pts',(-0.813879110112111,-0.498125538648156,
4.26606827749635));
#8615=CARTESIAN_POINT('Ctrl Pts',(-0.420960341352675,-0.883784830320034,
4.29448506591828));
#8616=CARTESIAN_POINT('Ctrl Pts',(0.224789069817019,-0.981132664539065,
4.32698303203636));
#8617=CARTESIAN_POINT('Ctrl Pts',(0.833681922437495,-0.56650552027897,4.36357743712977));
#8618=CARTESIAN_POINT('Ctrl Pts',(0.997525969733803,0.151809280111847,4.40021093558096));
#8619=CARTESIAN_POINT('Ctrl Pts',(0.629053416259707,0.790872367938504,4.43688813066444));
#8620=CARTESIAN_POINT('Ctrl Pts',(-0.0776376842752591,1.00903081883449,
4.47361454615104));
#8621=CARTESIAN_POINT('Ctrl Pts',(-0.669159294915032,0.723239602156119,
4.50630883475876));
#8622=CARTESIAN_POINT('Ctrl Pts',(-0.933615302724183,0.235422240437012,
4.53495405715562));
#8623=CARTESIAN_POINT('Ctrl Pts',(-0.933641466162531,-0.239764602920034,
4.55953364433428));
#8624=CARTESIAN_POINT('Ctrl Pts',(-0.706144252215777,-0.65830114813711,
4.58414298960005));
#8625=CARTESIAN_POINT('Ctrl Pts',(-0.305568054713619,-0.916660441466946,
4.60878302433065));
#8626=CARTESIAN_POINT('Ctrl Pts',(0.170387676510673,-0.952765931836802,
4.63345394982545));
#8627=CARTESIAN_POINT('Ctrl Pts',(0.542555110244804,-0.784634851727257,
4.65455753095455));
#8628=CARTESIAN_POINT('Ctrl Pts',(0.770225790729519,-0.54331566877176,4.67207538305286));
#8629=CARTESIAN_POINT('Ctrl Pts',(0.932090725649148,-0.231113115898143,
4.69063876644602));
#8630=CARTESIAN_POINT('Ctrl Pts',(0.957871337899541,0.221285409072723,4.71387291471119));
#8631=CARTESIAN_POINT('Ctrl Pts',(0.694319442459975,0.698311633436892,4.74180038845792));
#8632=CARTESIAN_POINT('Ctrl Pts',(0.216737061340996,0.962418705490843,4.76977721937668));
#8633=CARTESIAN_POINT('Ctrl Pts',(-0.329241357561265,0.931920409055914,
4.79780471923481));
#8634=CARTESIAN_POINT('Ctrl Pts',(-0.776106758281407,0.615017342938231,
4.82588478924082));
#8635=CARTESIAN_POINT('Ctrl Pts',(-0.986303575858324,0.107968492198592,
4.85401898069626));
#8636=CARTESIAN_POINT('Ctrl Pts',(-0.894329856751629,-0.434269986929119,
4.8822089287795));
#8637=CARTESIAN_POINT('Ctrl Pts',(-0.527226968394228,-0.845299850272977,
4.91045615450255));
#8638=CARTESIAN_POINT('Ctrl Pts',(0.0033919611434381,-0.998340479227608,
4.93876214814565));
#8639=CARTESIAN_POINT('Ctrl Pts',(0.535231960194268,-0.845295789931832,
4.96712834313108));
#8640=CARTESIAN_POINT('Ctrl Pts',(0.904933168151654,-0.431859589715681,
4.9955561182682));
#8641=CARTESIAN_POINT('Ctrl Pts',(0.998215666603856,0.116109753255343,5.02404679691162));
#8642=CARTESIAN_POINT('Ctrl Pts',(0.785186438599943,0.630876060238445,5.0526016457263));
#8643=CARTESIAN_POINT('Ctrl Pts',(0.329897474700307,0.954144141946419,5.0812218763083));
#8644=CARTESIAN_POINT('Ctrl Pts',(-0.22889329357451,0.985708576145502,5.10990864545268));
#8645=CARTESIAN_POINT('Ctrl Pts',(-0.719987155661827,0.714505791718518,
5.13866303733357));
#8646=CARTESIAN_POINT('Ctrl Pts',(-0.992173120872884,0.222413780858762,
5.16748611276041));
#8647=CARTESIAN_POINT('Ctrl Pts',(-0.960763757484564,-0.340411422023257,
5.19637880363374));
#8648=CARTESIAN_POINT('Ctrl Pts',(-0.633940084188984,-0.80142093923978,
5.22534214530267));
#8649=CARTESIAN_POINT('Ctrl Pts',(-0.110673692443478,-1.01836625645358,
5.25437676792106));
#8650=CARTESIAN_POINT('Ctrl Pts',(0.449182451185127,-0.923606231726753,
5.28348405622099));
#8651=CARTESIAN_POINT('Ctrl Pts',(0.873798643905496,-0.544251784946238,
5.31266356415371));
#8652=CARTESIAN_POINT('Ctrl Pts',(0.979170353153057,-0.17920951900525,5.33216668867801));
#8653=CARTESIAN_POINT('Ctrl Pts',(0.979195073394965,0.00441873155204175,
5.34192797255006));
#8654=CARTESIAN_POINT('Ctrl Pts',(1.08383455515366,-0.00100513229999224,
2.09412075287127));
#8655=CARTESIAN_POINT('Ctrl Pts',(1.0838072186452,0.202057385077309,2.10491512067412));
#8656=CARTESIAN_POINT('Ctrl Pts',(0.967176636812093,0.606569610116454,2.12652636292198));
#8657=CARTESIAN_POINT('Ctrl Pts',(0.496066254774699,1.02763200736581,2.15890649001074));
#8658=CARTESIAN_POINT('Ctrl Pts',(-0.126357494462602,1.13317581705174,2.19127042803801));
#8659=CARTESIAN_POINT('Ctrl Pts',(-0.709205564145551,0.891686385254436,
2.22360804916189));
#8660=CARTESIAN_POINT('Ctrl Pts',(-1.0739333900271,0.377472593954113,2.25592086261441));
#8661=CARTESIAN_POINT('Ctrl Pts',(-1.10916844440495,-0.251400260581686,
2.28820514288567));
#8662=CARTESIAN_POINT('Ctrl Pts',(-0.804703166881614,-0.802127600795733,
2.32045953364164));
#8663=CARTESIAN_POINT('Ctrl Pts',(-0.254453640242555,-1.10613142625631,
2.35268161694683));
#8664=CARTESIAN_POINT('Ctrl Pts',(0.372524133280107,-1.07084797948588,2.38486953313084));
#8665=CARTESIAN_POINT('Ctrl Pts',(0.884048629344189,-0.707746783112836,
2.4170211098838));
#8666=CARTESIAN_POINT('Ctrl Pts',(1.12368139865338,-0.128967810912809,2.44913462963003));
#8667=CARTESIAN_POINT('Ctrl Pts',(1.01879159895331,0.488100661391317,2.48120765737687));
#8668=CARTESIAN_POINT('Ctrl Pts',(0.671592645081585,0.875945276774875,2.50790086584788));
#8669=CARTESIAN_POINT('Ctrl Pts',(0.30248923948297,1.04055255032915,2.52923217303823));
#8670=CARTESIAN_POINT('Ctrl Pts',(0.00273063932233121,1.08299928584134,
2.54521959464766));
#8671=CARTESIAN_POINT('Ctrl Pts',(-0.296918707076225,1.04061966320984,2.56119554297854));
#8672=CARTESIAN_POINT('Ctrl Pts',(-0.57295347024857,0.917140579769783,2.57715977596269));
#8673=CARTESIAN_POINT('Ctrl Pts',(-0.803692754746948,0.722157016036992,
2.59311219792725));
#8674=CARTESIAN_POINT('Ctrl Pts',(-1.0152363324343,0.406108796017378,2.61318476146475));
#8675=CARTESIAN_POINT('Ctrl Pts',(-1.08983178300628,0.037250869792953,2.63264744709217));
#8676=CARTESIAN_POINT('Ctrl Pts',(-1.02750791393542,-0.31367372199185,2.65149873120761));
#8677=CARTESIAN_POINT('Ctrl Pts',(-0.881447705942929,-0.638275149283354,
2.67033658335757));
#8678=CARTESIAN_POINT('Ctrl Pts',(-0.555598070387777,-0.956318325625562,
2.69385882342524));
#8679=CARTESIAN_POINT('Ctrl Pts',(-0.0892637312173702,-1.08706975249208,
2.71891053244989));
#8680=CARTESIAN_POINT('Ctrl Pts',(0.441231110674361,-1.0120947255311,2.74705695241423));
#8681=CARTESIAN_POINT('Ctrl Pts',(0.887695511526617,-0.680828785898897,
2.77515950943379));
#8682=CARTESIAN_POINT('Ctrl Pts',(1.09296623655105,-0.112574626725122,2.80632510595015));
#8683=CARTESIAN_POINT('Ctrl Pts',(1.01238753003802,0.422468371144573,2.83432700014897));
#8684=CARTESIAN_POINT('Ctrl Pts',(0.685489237407475,0.854090959271124,2.86228097985869));
#8685=CARTESIAN_POINT('Ctrl Pts',(0.24818119515735,1.0509253589982,2.88708521506922));
#8686=CARTESIAN_POINT('Ctrl Pts',(-0.281912505533628,1.05574552847318,2.91494833111401));
#8687=CARTESIAN_POINT('Ctrl Pts',(-0.849831183761748,0.754692758675727,
2.94739661399269));
#8688=CARTESIAN_POINT('Ctrl Pts',(-1.14444668157779,0.00348830941917116,
2.98746544745627));
#8689=CARTESIAN_POINT('Ctrl Pts',(-0.838821075659442,-0.773323040553238,
3.02895622562989));
#8690=CARTESIAN_POINT('Ctrl Pts',(-0.0887510849550236,-1.13418240132233,
3.0703256506113));
#8691=CARTESIAN_POINT('Ctrl Pts',(0.704252876635555,-0.88910978446688,3.11157120272713));
#8692=CARTESIAN_POINT('Ctrl Pts',(1.11741889612126,-0.172268714907602,3.15269084027887));
#8693=CARTESIAN_POINT('Ctrl Pts',(0.933635635982071,0.631579498941108,3.19368244226885));
#8694=CARTESIAN_POINT('Ctrl Pts',(0.253516921328693,1.09472482298316,3.23454449498551));
#8695=CARTESIAN_POINT('Ctrl Pts',(-0.46578270941342,0.984823889831234,3.27074921367188));
#8696=CARTESIAN_POINT('Ctrl Pts',(-0.902683215290603,0.556363270548466,
3.30234310258505));
#8697=CARTESIAN_POINT('Ctrl Pts',(-1.05697667075416,0.05735687056592,3.32936366304358));
#8698=CARTESIAN_POINT('Ctrl Pts',(-0.953160259240073,-0.454456668822736,
3.35632572854271));
#8699=CARTESIAN_POINT('Ctrl Pts',(-0.655710111295285,-0.807878038485106,
3.38023751987761));
#8700=CARTESIAN_POINT('Ctrl Pts',(-0.197041480200333,-1.03414796641898,
3.40708995144052));
#8701=CARTESIAN_POINT('Ctrl Pts',(0.273086892424193,-1.01475766405274,3.43090374642035));
#8702=CARTESIAN_POINT('Ctrl Pts',(0.758645088847692,-0.723565062091646,
3.46060506771804));
#8703=CARTESIAN_POINT('Ctrl Pts',(1.02619655264658,-0.268984419353583,3.4872756034617));
#8704=CARTESIAN_POINT('Ctrl Pts',(0.996387322687455,0.303025364684566,3.51683147442567));
#8705=CARTESIAN_POINT('Ctrl Pts',(0.728951561944792,0.740953674049451,3.54337068720782));
#8706=CARTESIAN_POINT('Ctrl Pts',(0.285110217835692,0.996730445071976,3.56984942607481));
#8707=CARTESIAN_POINT('Ctrl Pts',(-0.311384544736447,1.01283968272107,3.60067110558919));
#8708=CARTESIAN_POINT('Ctrl Pts',(-0.895518055039455,0.615482305648,3.6357943259958));
#8709=CARTESIAN_POINT('Ctrl Pts',(-1.0409159420416,-0.0283394110497346,
3.66860908547933));
#8710=CARTESIAN_POINT('Ctrl Pts',(-0.874227166910078,-0.499830766853547,
3.6947954969822));
#8711=CARTESIAN_POINT('Ctrl Pts',(-0.630592962401571,-0.783616493190624,
3.71440219407833));
#8712=CARTESIAN_POINT('Ctrl Pts',(-0.300015163190702,-0.957974480984689,
3.73397463201407));
#8713=CARTESIAN_POINT('Ctrl Pts',(0.111783740171799,-1.00466671708127,3.75568519526895));
#8714=CARTESIAN_POINT('Ctrl Pts',(0.548934143160709,-0.857711337819638,
3.77951940523228));
#8715=CARTESIAN_POINT('Ctrl Pts',(0.890168052144742,-0.489407069594645,
3.8054635732035));
#8716=CARTESIAN_POINT('Ctrl Pts',(0.983967638561348,-0.120456653152492,
3.82514559136655));
#8717=CARTESIAN_POINT('Ctrl Pts',(0.966063153040552,0.132090193079272,3.83860912181926));
#8718=CARTESIAN_POINT('Ctrl Pts',(0.928032981075702,0.310180874839214,3.84829683488476));
#8719=CARTESIAN_POINT('Ctrl Pts',(0.79732422491957,0.603293178112202,3.86523401611496));
#8720=CARTESIAN_POINT('Ctrl Pts',(0.446210687994022,0.917210804455452,3.88938327655937));
#8721=CARTESIAN_POINT('Ctrl Pts',(-0.110068761338206,1.01148074075704,3.91829259262403));
#8722=CARTESIAN_POINT('Ctrl Pts',(-0.629778714922221,0.795980055673373,
3.9471315659034));
#8723=CARTESIAN_POINT('Ctrl Pts',(-0.954492360839048,0.338049134353879,
3.9759016731882));
#8724=CARTESIAN_POINT('Ctrl Pts',(-0.985690335581518,-0.221102775015846,
4.00460364145414));
#8725=CARTESIAN_POINT('Ctrl Pts',(-0.71527423954657,-0.710019115305869,
4.0332386406658));
#8726=CARTESIAN_POINT('Ctrl Pts',(-0.22730521254799,-0.979503584524682,
4.0618077501134));
#8727=CARTESIAN_POINT('Ctrl Pts',(0.327979039642183,-0.948145702873503,
4.09031217793584));
#8728=CARTESIAN_POINT('Ctrl Pts',(0.780465135736674,-0.626881939976658,
4.1187531685785));
#8729=CARTESIAN_POINT('Ctrl Pts',(0.992203650298369,-0.115250509294351,
4.14713201945934));
#8730=CARTESIAN_POINT('Ctrl Pts',(0.899499190924821,0.429452598894815,4.17545011398173));
#8731=CARTESIAN_POINT('Ctrl Pts',(0.531938608728281,0.840456211956105,4.20370881077333));
#8732=CARTESIAN_POINT('Ctrl Pts',(0.00320558862913967,0.992645561888121,
4.23190968257249));
#8733=CARTESIAN_POINT('Ctrl Pts',(-0.524589061186669,0.840384906564921,
4.26005395738908));
#8734=CARTESIAN_POINT('Ctrl Pts',(-0.875886060224354,0.446832139458484,
4.28710339665259));
#8735=CARTESIAN_POINT('Ctrl Pts',(-0.975392699171194,-0.0461734306504795,
4.31306524464901));
#8736=CARTESIAN_POINT('Ctrl Pts',(-0.833014281038782,-0.505523598165439,
4.33795023099546));
#8737=CARTESIAN_POINT('Ctrl Pts',(-0.432085868110668,-0.898848002117052,
4.36693537151759));
#8738=CARTESIAN_POINT('Ctrl Pts',(0.224988129031288,-0.997494004660513,
4.39999650828921));
#8739=CARTESIAN_POINT('Ctrl Pts',(0.842309514128291,-0.576595861558382,
4.43710735610631));
#8740=CARTESIAN_POINT('Ctrl Pts',(1.00752258942579,0.149768590973636,4.47414020946719));
#8741=CARTESIAN_POINT('Ctrl Pts',(0.635768391948925,0.793634591411079,4.51110029373353));
#8742=CARTESIAN_POINT('Ctrl Pts',(-0.0743383737232185,1.01237269509007,
4.54799164202132));
#8743=CARTESIAN_POINT('Ctrl Pts',(-0.666508256149446,0.725845969874338,
4.58072644727242));
#8744=CARTESIAN_POINT('Ctrl Pts',(-0.930500361436642,0.238581639159787,
4.60933197480601));
#8745=CARTESIAN_POINT('Ctrl Pts',(-0.930395932628208,-0.235017133168795,
4.63382810381776));
#8746=CARTESIAN_POINT('Ctrl Pts',(-0.704048414868301,-0.651201238468357,
4.65829980147231));
#8747=CARTESIAN_POINT('Ctrl Pts',(-0.306457717371693,-0.90747432123094,
4.68274942071083));
#8748=CARTESIAN_POINT('Ctrl Pts',(0.164900848925934,-0.943116217052762,
4.70718032224016));
#8749=CARTESIAN_POINT('Ctrl Pts',(0.532586291489543,-0.7768743398517,4.72802875324737));
#8750=CARTESIAN_POINT('Ctrl Pts',(0.757186657608633,-0.538773046044311,
4.7453112080288));
#8751=CARTESIAN_POINT('Ctrl Pts',(0.916668695103853,-0.231094170555637,
4.76360306157553));
#8752=CARTESIAN_POINT('Ctrl Pts',(0.941879012311262,0.213904287027886,4.78645305810177));
#8753=CARTESIAN_POINT('Ctrl Pts',(0.683080673189071,0.681957662619039,4.81385719170469));
#8754=CARTESIAN_POINT('Ctrl Pts',(0.215392937090561,0.940387267485015,4.84124578391745));
#8755=CARTESIAN_POINT('Ctrl Pts',(-0.317945518562309,0.91042074411468,4.86862180210215));
#8756=CARTESIAN_POINT('Ctrl Pts',(-0.753387179512403,0.601407580332747,
4.89598712456847));
#8757=CARTESIAN_POINT('Ctrl Pts',(-0.957643715091763,0.108246828535003,
4.92334415364639));
#8758=CARTESIAN_POINT('Ctrl Pts',(-0.868233611205659,-0.417881537488712,
4.95069508929941));
#8759=CARTESIAN_POINT('Ctrl Pts',(-0.512669209156949,-0.815746003186908,
4.97804224075945));
#8760=CARTESIAN_POINT('Ctrl Pts',(4.31839669338944E-5,-0.963454107947432,
5.00538786962271));
#8761=CARTESIAN_POINT('Ctrl Pts',(0.512769332970879,-0.815744639868486,
5.03273427529492));
#8762=CARTESIAN_POINT('Ctrl Pts',(0.868364986197536,-0.417849081119337,
5.06008373717176));
#8763=CARTESIAN_POINT('Ctrl Pts',(0.957786283176147,0.108348086643308,5.08743854354636));
#8764=CARTESIAN_POINT('Ctrl Pts',(0.753496435761779,0.601605495981712,5.11480096457011));
#8765=CARTESIAN_POINT('Ctrl Pts',(0.317936353225337,0.910686321698448,5.1421732876434));
#8766=CARTESIAN_POINT('Ctrl Pts',(-0.215540765577659,0.940677697820739,
5.16955775201152));
#8767=CARTESIAN_POINT('Ctrl Pts',(-0.683455937250816,0.682116790417354,
5.19695665459153));
#8768=CARTESIAN_POINT('Ctrl Pts',(-0.942253548854584,0.213950549125594,
5.22437212570714));
#8769=CARTESIAN_POINT('Ctrl Pts',(-0.912297345239954,-0.320500930766703,
5.25180662638367));
#8770=CARTESIAN_POINT('Ctrl Pts',(-0.602362624559855,-0.757478419318723,
5.27926181463212));
#8771=CARTESIAN_POINT('Ctrl Pts',(-0.107056118750729,-0.962692795935569,
5.30674105031171));
#8772=CARTESIAN_POINT('Ctrl Pts',(0.421984195787826,-0.873059479070634,
5.33424381353539));
#8773=CARTESIAN_POINT('Ctrl Pts',(0.822562701518577,-0.514974705783212,
5.36177808819317));
#8774=CARTESIAN_POINT('Ctrl Pts',(0.921747231678515,-0.171138641059886,
5.38014514248733));
#8775=CARTESIAN_POINT('Ctrl Pts',(0.921770527134554,0.00190593732143055,
5.38934382105108));
#8776=CARTESIAN_POINT('Ctrl Pts',(1.06702201959591,0.00285043970073984,
2.0215475585234));
#8777=CARTESIAN_POINT('Ctrl Pts',(1.06699508957157,0.202893489956048,2.03218141793157));
#8778=CARTESIAN_POINT('Ctrl Pts',(0.952197003975437,0.601527586454393,2.05347419254553));
#8779=CARTESIAN_POINT('Ctrl Pts',(0.487056211644658,1.01753294235621,2.08545253086904));
#8780=CARTESIAN_POINT('Ctrl Pts',(-0.128863848342645,1.1221315680947,2.11747652423528));
#8781=CARTESIAN_POINT('Ctrl Pts',(-0.706907658382305,0.882825885801358,
2.14954193386969));
#8782=CARTESIAN_POINT('Ctrl Pts',(-1.06947298146975,0.371955511405459,2.18164790285542));
#8783=CARTESIAN_POINT('Ctrl Pts',(-1.10473354554263,-0.254222576858051,
2.21379199658814));
#8784=CARTESIAN_POINT('Ctrl Pts',(-0.801098332840217,-0.803816818903664,
2.24597243091371));
#8785=CARTESIAN_POINT('Ctrl Pts',(-0.251022866900719,-1.107928868166,2.27818709518381));
#8786=CARTESIAN_POINT('Ctrl Pts',(0.377157547542421,-1.07275865606352,2.31043394078));
#8787=CARTESIAN_POINT('Ctrl Pts',(0.890814984617286,-0.708364377644769,
2.34271091875739));
#8788=CARTESIAN_POINT('Ctrl Pts',(1.13206003543397,-0.12616681018466,2.37501578311069));
#8789=CARTESIAN_POINT('Ctrl Pts',(1.02649991184449,0.495927285016085,2.4073466493677));
#8790=CARTESIAN_POINT('Ctrl Pts',(0.675888865904133,0.887802847820554,2.43430832444967));
#8791=CARTESIAN_POINT('Ctrl Pts',(0.302465182735742,1.05436962634722,2.45588912818849));
#8792=CARTESIAN_POINT('Ctrl Pts',(-0.00110925844173351,1.09737681688059,
2.47207972994715));
#8793=CARTESIAN_POINT('Ctrl Pts',(-0.304888662325547,1.05443550943871,2.48827516246545));
#8794=CARTESIAN_POINT('Ctrl Pts',(-0.585016322460578,0.929148428211227,
2.50447514794601));
#8795=CARTESIAN_POINT('Ctrl Pts',(-0.819419308229265,0.731096076322071,
2.52067935421188));
#8796=CARTESIAN_POINT('Ctrl Pts',(-1.03454937622517,0.409738788275447,2.5410898548685));
#8797=CARTESIAN_POINT('Ctrl Pts',(-1.110579327663,0.0341785358218987,2.56090566398939));
#8798=CARTESIAN_POINT('Ctrl Pts',(-1.04705118956169,-0.3236433791638,2.5801267491674));
#8799=CARTESIAN_POINT('Ctrl Pts',(-0.898010236343792,-0.654911589195166,
2.59935087157429));
#8800=CARTESIAN_POINT('Ctrl Pts',(-0.565109570799394,-0.97997251636004,
2.62338602717653));
#8801=CARTESIAN_POINT('Ctrl Pts',(-0.0877645744898903,-1.11391907054818,
2.6490300997342));
#8802=CARTESIAN_POINT('Ctrl Pts',(0.456080346993929,-1.03711194963536,2.67788419010735));
#8803=CARTESIAN_POINT('Ctrl Pts',(0.914673548406407,-0.697098327564633,
2.70674252653505));
#8804=CARTESIAN_POINT('Ctrl Pts',(1.12602774396051,-0.112418131739695,2.73881013194141));
#8805=CARTESIAN_POINT('Ctrl Pts',(1.04307840629854,0.439074671072632,2.76767167730267));
#8806=CARTESIAN_POINT('Ctrl Pts',(0.705668036928256,0.884771411857633,2.79653215624472));
#8807=CARTESIAN_POINT('Ctrl Pts',(0.253455787403711,1.08841958876369,2.82218366694516));
#8808=CARTESIAN_POINT('Ctrl Pts',(-0.295493024176249,1.09346191224925,2.85103797378248));
#8809=CARTESIAN_POINT('Ctrl Pts',(-0.884664851586657,0.781403855485988,
2.88469536651339));
#8810=CARTESIAN_POINT('Ctrl Pts',(-1.19129978902031,0.000581549421014766,
2.92635152585855));
#8811=CARTESIAN_POINT('Ctrl Pts',(-0.873168334733573,-0.809044188315319,
2.96958770031669));
#8812=CARTESIAN_POINT('Ctrl Pts',(-0.08991365677559,-1.18627345200091,3.01279661748751));
#8813=CARTESIAN_POINT('Ctrl Pts',(0.740303848481622,-0.930075865252766,
3.05597296819526));
#8814=CARTESIAN_POINT('Ctrl Pts',(1.17404659392292,-0.178225554833157,3.09911149645123));
#8815=CARTESIAN_POINT('Ctrl Pts',(0.981161351803577,0.666927533936675,3.14220724582939));
#8816=CARTESIAN_POINT('Ctrl Pts',(0.264871552947168,1.15510320472919,3.18525471062778));
#8817=CARTESIAN_POINT('Ctrl Pts',(-0.494428740123167,1.03935387427447,3.2234727638888));
#8818=CARTESIAN_POINT('Ctrl Pts',(-0.956404802565376,0.586449571383587,
3.25687471171129));
#8819=CARTESIAN_POINT('Ctrl Pts',(-1.11979346868318,0.058258331371253,3.28547881446806));
#8820=CARTESIAN_POINT('Ctrl Pts',(-1.00986054768212,-0.484166937058073,
3.31405254369003));
#8821=CARTESIAN_POINT('Ctrl Pts',(-0.694283302029937,-0.859206449360406,
3.33942674184122));
#8822=CARTESIAN_POINT('Ctrl Pts',(-0.20720327925374,-1.09954269454893,3.36794392261175));
#8823=CARTESIAN_POINT('Ctrl Pts',(0.29265908786554,-1.07902180486329,3.39326606792902));
#8824=CARTESIAN_POINT('Ctrl Pts',(0.809475546507311,-0.769138857714769,
3.42487917029462));
#8825=CARTESIAN_POINT('Ctrl Pts',(1.09462539138736,-0.28487361877622,3.45329625277239));
#8826=CARTESIAN_POINT('Ctrl Pts',(1.06291369715779,0.325256037101083,3.48482268248564));
#8827=CARTESIAN_POINT('Ctrl Pts',(0.777434815872461,0.7928386116761,3.5131592168709));
#8828=CARTESIAN_POINT('Ctrl Pts',(0.303177481860876,1.06621189571728,3.54145653166712));
#8829=CARTESIAN_POINT('Ctrl Pts',(-0.334758663253051,1.0835070513843,3.57442250475897));
#8830=CARTESIAN_POINT('Ctrl Pts',(-0.960229074971341,0.658229837595933,
3.61202995640657));
#8831=CARTESIAN_POINT('Ctrl Pts',(-1.11619274136482,-0.0318103647610028,
3.64720653123438));
#8832=CARTESIAN_POINT('Ctrl Pts',(-0.937428906276688,-0.537533778848072,
3.67529509327478));
#8833=CARTESIAN_POINT('Ctrl Pts',(-0.676001017110024,-0.84206151951191,
3.69633537325015));
#8834=CARTESIAN_POINT('Ctrl Pts',(-0.321092341582353,-1.02926596955437,
3.7173506245525));
#8835=CARTESIAN_POINT('Ctrl Pts',(0.121208828079285,-1.07942774678667,3.74067104000155));
#8836=CARTESIAN_POINT('Ctrl Pts',(0.590969798913608,-0.921535378852899,
3.76628537873098));
#8837=CARTESIAN_POINT('Ctrl Pts',(0.957844459619203,-0.525614588470272,
3.79417761398359));
#8838=CARTESIAN_POINT('Ctrl Pts',(1.05876459652488,-0.12875481310516,3.81535214818028));
#8839=CARTESIAN_POINT('Ctrl Pts',(1.0395064635086,0.142927269520196,3.82983622592237));
#8840=CARTESIAN_POINT('Ctrl Pts',(0.998590856068431,0.334531305443016,3.84025938000999));
#8841=CARTESIAN_POINT('Ctrl Pts',(0.857941964811768,0.649944025822184,3.85848631113206));
#8842=CARTESIAN_POINT('Ctrl Pts',(0.479993992774951,0.987881570361023,3.88448594098035));
#8843=CARTESIAN_POINT('Ctrl Pts',(-0.118980327541849,1.08940918853345,3.91561757288294));
#8844=CARTESIAN_POINT('Ctrl Pts',(-0.678729907854082,0.85733025713029,3.94668180840835));
#8845=CARTESIAN_POINT('Ctrl Pts',(-1.02852647823543,0.364047032000577,3.97767703233711));
#8846=CARTESIAN_POINT('Ctrl Pts',(-1.06214407322819,-0.238348644573769,
4.0086026043394));
#8847=CARTESIAN_POINT('Ctrl Pts',(-0.770799167454087,-0.765104131388401,
4.03945751410833));
#8848=CARTESIAN_POINT('Ctrl Pts',(-0.24506993964978,-1.05543488480932,4.07024098687146));
#8849=CARTESIAN_POINT('Ctrl Pts',(0.353129677630186,-1.02164169574851,4.10095223014905));
#8850=CARTESIAN_POINT('Ctrl Pts',(0.840502862789607,-0.675586766930572,
4.13159054166329));
#8851=CARTESIAN_POINT('Ctrl Pts',(1.06850001744841,-0.124608973291446,4.16215528527946));
#8852=CARTESIAN_POINT('Ctrl Pts',(0.968667539921783,0.461800789232989,4.19264586113681));
#8853=CARTESIAN_POINT('Ctrl Pts',(0.573075375497625,0.904095810892864,4.22306181606733));
#8854=CARTESIAN_POINT('Ctrl Pts',(0.00428398543883978,1.06777175324867,
4.25340259677658));
#8855=CARTESIAN_POINT('Ctrl Pts',(-0.563191060635299,0.904009958454533,
4.28366811821645));
#8856=CARTESIAN_POINT('Ctrl Pts',(-0.940669220907235,0.481061734634649,
4.31273939615205));
#8857=CARTESIAN_POINT('Ctrl Pts',(-1.04748681672637,-0.0484309683621674,
4.34062676179975));
#8858=CARTESIAN_POINT('Ctrl Pts',(-0.894659216501438,-0.541420541857352,
4.3673360049139));
#8859=CARTESIAN_POINT('Ctrl Pts',(-0.464581269885186,-0.963235408380499,
4.39842750092416));
#8860=CARTESIAN_POINT('Ctrl Pts',(0.239565566362356,-1.06883033579405,4.43386078841037));
#8861=CARTESIAN_POINT('Ctrl Pts',(0.900207301627467,-0.6181471938036,4.4735881815693));
#8862=CARTESIAN_POINT('Ctrl Pts',(1.07661736077248,0.158307456468171,4.51318028163458));
#8863=CARTESIAN_POINT('Ctrl Pts',(0.679619107697134,0.845445051684285,4.55263682700741));
#8864=CARTESIAN_POINT('Ctrl Pts',(-0.0772188720163175,1.07831123772824,
4.59195908839367));
#8865=CARTESIAN_POINT('Ctrl Pts',(-0.707169488136082,0.773252871890353,
4.62679420162289));
#8866=CARTESIAN_POINT('Ctrl Pts',(-0.987518254466977,0.255555062644542,
4.65718831119431));
#8867=CARTESIAN_POINT('Ctrl Pts',(-0.987344296695494,-0.246928877186952,
4.68318021964439));
#8868=CARTESIAN_POINT('Ctrl Pts',(-0.747395974394147,-0.68790253874418,
4.70911509298375));
#8869=CARTESIAN_POINT('Ctrl Pts',(-0.326598919534621,-0.959047210599774,
4.73499264228026));
#8870=CARTESIAN_POINT('Ctrl Pts',(0.171526528910553,-0.996613146528814,
4.76081164773556));
#8871=CARTESIAN_POINT('Ctrl Pts',(0.559559675319348,-0.821106466207549,
4.78282032257176));
#8872=CARTESIAN_POINT('Ctrl Pts',(0.796278934310142,-0.570126029209407,
4.80103769428559));
#8873=CARTESIAN_POINT('Ctrl Pts',(0.964224236533784,-0.246079960768308,
4.82030349152749));
#8874=CARTESIAN_POINT('Ctrl Pts',(0.990634981866468,0.222032268895686,4.84434428541031));
#8875=CARTESIAN_POINT('Ctrl Pts',(0.718768909207029,0.713425976685633,4.87312285291378));
#8876=CARTESIAN_POINT('Ctrl Pts',(0.228511728246258,0.984171670659741,4.90183375867155));
#8877=CARTESIAN_POINT('Ctrl Pts',(-0.329439271525028,0.952675739973614,
4.93047742700953));
#8878=CARTESIAN_POINT('Ctrl Pts',(-0.784025344868638,0.629894027325748,
4.95905533359007));
#8879=CARTESIAN_POINT('Ctrl Pts',(-0.996744501476427,0.115900336236449,
4.98756854278546));
#8880=CARTESIAN_POINT('Ctrl Pts',(-0.903599797834191,-0.431268663631399,
5.01601837689846));
#8881=CARTESIAN_POINT('Ctrl Pts',(-0.534433841777186,-0.844113612462787,
5.04440611789283));
#8882=CARTESIAN_POINT('Ctrl Pts',(-0.00334246362797946,-0.996947925202839,
5.07273313603078));
#8883=CARTESIAN_POINT('Ctrl Pts',(0.526547243855696,-0.844122845511364,
5.10100084493586));
#8884=CARTESIAN_POINT('Ctrl Pts',(0.893161693859534,-0.433647847012934,
5.12921071114398));
#8885=CARTESIAN_POINT('Ctrl Pts',(0.985017050564764,0.107878463430296,5.15736425383812));
#8886=CARTESIAN_POINT('Ctrl Pts',(0.775096210047194,0.614286586251671,5.1854630337029));
#8887=CARTESIAN_POINT('Ctrl Pts',(0.328772572338644,0.930794298175775,5.21350867924155));
#8888=CARTESIAN_POINT('Ctrl Pts',(-0.216531421468218,0.961276383482143,
5.24150282972688));
#8889=CARTESIAN_POINT('Ctrl Pts',(-0.693626467566039,0.697442197976963,
5.26944723759027));
#8890=CARTESIAN_POINT('Ctrl Pts',(-0.956780044053587,0.221028354809448,
5.29734354491797));
#8891=CARTESIAN_POINT('Ctrl Pts',(-0.926194208137696,-0.321458272100224,
5.3251937796117));
#8892=CARTESIAN_POINT('Ctrl Pts',(-0.612185879018724,-0.763866525937045,
5.35299922629289));
#8893=CARTESIAN_POINT('Ctrl Pts',(-0.111725843695108,-0.971021766407051,
5.38076291905228));
#8894=CARTESIAN_POINT('Ctrl Pts',(0.421454260882621,-0.880515937840451,
5.40848407795733));
#8895=CARTESIAN_POINT('Ctrl Pts',(0.824100639480779,-0.520346924625745,
5.43617046078395));
#8896=CARTESIAN_POINT('Ctrl Pts',(0.92351355797063,-0.17546039163511,5.45459465534717));
#8897=CARTESIAN_POINT('Ctrl Pts',(0.923536902282142,-0.00205290235935909,
5.46381262547553));
#8898=CARTESIAN_POINT('Ctrl Pts',(1.02243941136618,0.00398423891480934,
2.00010574185718));
#8899=CARTESIAN_POINT('Ctrl Pts',(1.02241359427953,0.195760105709546,2.01030013552781));
#8900=CARTESIAN_POINT('Ctrl Pts',(0.912384794808815,0.57783074171643,2.03070887226764));
#8901=CARTESIAN_POINT('Ctrl Pts',(0.466210030566678,0.976979667346393,2.06138810717927));
#8902=CARTESIAN_POINT('Ctrl Pts',(-0.125096972995613,1.07745189775172,2.09213285468625));
#8903=CARTESIAN_POINT('Ctrl Pts',(-0.680513135833094,0.847598882016436,
2.1229425677617));
#8904=CARTESIAN_POINT('Ctrl Pts',(-1.02921948039241,0.35639070652297,2.15381627278417));
#8905=CARTESIAN_POINT('Ctrl Pts',(-1.06323558233127,-0.246247511674403,
2.18475313583275));
#8906=CARTESIAN_POINT('Ctrl Pts',(-0.770826846999395,-0.77569409414987,
2.21575219104532));
#8907=CARTESIAN_POINT('Ctrl Pts',(-0.240514282436741,-1.06897711434002,
2.24681248125642));
#8908=CARTESIAN_POINT('Ctrl Pts',(0.365719763837382,-1.03512322488853,2.27793292555432));
#8909=CARTESIAN_POINT('Ctrl Pts',(0.861960816498296,-0.683194362032242,
2.30911251383287));
#8910=CARTESIAN_POINT('Ctrl Pts',(1.09531889997021,-0.120271361501286,2.34034991634459));
#8911=CARTESIAN_POINT('Ctrl Pts',(0.993237192117574,0.481895386113469,2.37164430422677));
#8912=CARTESIAN_POINT('Ctrl Pts',(0.653571524566261,0.861659412057779,2.39776861909535));
#8913=CARTESIAN_POINT('Ctrl Pts',(0.291454062137944,1.02320284426481,2.41869618695453));
#8914=CARTESIAN_POINT('Ctrl Pts',(-0.00308920568304123,1.06494358035969,
2.43440512380543));
#8915=CARTESIAN_POINT('Ctrl Pts',(-0.297997185345012,1.02327054546842,2.45012728658302));
#8916=CARTESIAN_POINT('Ctrl Pts',(-0.570097692954665,0.901588560504387,
2.46586256288552));
#8917=CARTESIAN_POINT('Ctrl Pts',(-0.797915324645491,0.709118942927343,
2.48161057136306));
#8918=CARTESIAN_POINT('Ctrl Pts',(-1.00712518371007,0.396636113599795,2.50145794064213));
#8919=CARTESIAN_POINT('Ctrl Pts',(-1.08116460684588,0.0311698313189306,
2.52074077270457));
#8920=CARTESIAN_POINT('Ctrl Pts',(-1.01930513653729,-0.317331812896037,
2.5394607174683));
#8921=CARTESIAN_POINT('Ctrl Pts',(-0.874086747019434,-0.640136090368379,
2.55819302267196));
#8922=CARTESIAN_POINT('Ctrl Pts',(-0.549496069959448,-0.957169806277918,
2.58163052088621));
#8923=CARTESIAN_POINT('Ctrl Pts',(-0.0835160615693929,-1.08799952729685,
2.6066640277496));
#8924=CARTESIAN_POINT('Ctrl Pts',(0.447882551085116,-1.01298309850681,2.6348572614683));
#8925=CARTESIAN_POINT('Ctrl Pts',(0.896526797653208,-0.680517624893238,
2.66308300818814));
#8926=CARTESIAN_POINT('Ctrl Pts',(1.10361806773707,-0.107914019055422,2.69448791650807));
#8927=CARTESIAN_POINT('Ctrl Pts',(1.02236526582386,0.43282548322369,2.72278440192714));
#8928=CARTESIAN_POINT('Ctrl Pts',(0.691233446933462,0.870356607176783,2.75111176990363));
#8929=CARTESIAN_POINT('Ctrl Pts',(0.246868968583059,1.07055085263004,2.77631849214705));
#8930=CARTESIAN_POINT('Ctrl Pts',(-0.293110275260041,1.07554167301612,2.80470081460215));
#8931=CARTESIAN_POINT('Ctrl Pts',(-0.873377993524284,0.768396352809485,
2.83784367708145));
#8932=CARTESIAN_POINT('Ctrl Pts',(-1.17608632993973,-0.00167480100091063,
2.87892742744357));
#8933=CARTESIAN_POINT('Ctrl Pts',(-0.862005440846571,-0.801794854597139,
2.92164667510429));
#8934=CARTESIAN_POINT('Ctrl Pts',(-0.0868001045588601,-1.17546983264539,
2.9644142252545));
#8935=CARTESIAN_POINT('Ctrl Pts',(0.736580981803708,-0.921694810107848,
3.00722624540655));
#8936=CARTESIAN_POINT('Ctrl Pts',(1.16774349960592,-0.174918209614478,3.05007784308638));
#8937=CARTESIAN_POINT('Ctrl Pts',(0.976072265924129,0.666290888680979,3.09296369279926));
#8938=CARTESIAN_POINT('Ctrl Pts',(0.262058174942946,1.15328967289916,3.13588034038676));
#8939=CARTESIAN_POINT('Ctrl Pts',(-0.496427378766351,1.03794803578382,3.17404809518878));
#8940=CARTESIAN_POINT('Ctrl Pts',(-0.958686700933804,0.584914097624343,
3.20746239375664));
#8941=CARTESIAN_POINT('Ctrl Pts',(-1.12243569410531,0.0559111282632584,
3.23610726859073));
#8942=CARTESIAN_POINT('Ctrl Pts',(-1.01225564720179,-0.488112652692135,
3.26476379086583));
#8943=CARTESIAN_POINT('Ctrl Pts',(-0.695487043547354,-0.864710880467027,
3.29023409387107));
#8944=CARTESIAN_POINT('Ctrl Pts',(-0.205898661278593,-1.10632076377313,
3.31889882744695));
#8945=CARTESIAN_POINT('Ctrl Pts',(0.297081287657339,-1.08581158838707,3.34437380568392));
#8946=CARTESIAN_POINT('Ctrl Pts',(0.817823747991888,-0.773631518006107,
3.37622271510012));
#8947=CARTESIAN_POINT('Ctrl Pts',(1.10559906046499,-0.285197856857749,3.40488530682305));
#8948=CARTESIAN_POINT('Ctrl Pts',(1.0736525234882,0.331169973155956,3.43673056973207));
#8949=CARTESIAN_POINT('Ctrl Pts',(0.784996582513853,0.804116540088881,3.46538534226499));
#8950=CARTESIAN_POINT('Ctrl Pts',(0.304802421955024,1.08099686803911,3.49403458049713));
#8951=CARTESIAN_POINT('Ctrl Pts',(-0.341944614013262,1.098636104481,3.52745168943803));
#8952=CARTESIAN_POINT('Ctrl Pts',(-0.977091025315939,0.667069718432036,
3.56562507555433));
#8953=CARTESIAN_POINT('Ctrl Pts',(-1.13595754845858,-0.034657215805678,
3.60139104564868));
#8954=CARTESIAN_POINT('Ctrl Pts',(-0.953933695872026,-0.549739668884208,
3.62999460912882));
#8955=CARTESIAN_POINT('Ctrl Pts',(-0.687479364990766,-0.860183893070429,
3.65144052291524));
#8956=CARTESIAN_POINT('Ctrl Pts',(-0.325442973517683,-1.05119495832465,
3.67287541516038));
#8957=CARTESIAN_POINT('Ctrl Pts',(0.126139312124764,-1.10245556695548,3.69668276834371));
#8958=CARTESIAN_POINT('Ctrl Pts',(0.606262182001061,-0.941165677336213,
3.72285638725491));
#8959=CARTESIAN_POINT('Ctrl Pts',(0.981703226798656,-0.536091933987129,
3.75139484192606));
#8960=CARTESIAN_POINT('Ctrl Pts',(1.08510429065794,-0.12966335831906,3.77307496323289));
#8961=CARTESIAN_POINT('Ctrl Pts',(1.06536235673658,0.148839679722951,3.78792185774525));
#8962=CARTESIAN_POINT('Ctrl Pts',(1.02340870619934,0.345313817801113,3.79860936295049));
#8963=CARTESIAN_POINT('Ctrl Pts',(0.879143926657432,0.668877663471392,3.81730516467634));
#8964=CARTESIAN_POINT('Ctrl Pts',(0.49119057265482,1.01587840437015,3.84399122167101));
#8965=CARTESIAN_POINT('Ctrl Pts',(-0.1244886820771,1.12034446949229,3.87598677430555));
#8966=CARTESIAN_POINT('Ctrl Pts',(-0.700571603791792,0.881592069567747,
3.90794936018184));
#8967=CARTESIAN_POINT('Ctrl Pts',(-1.06104856205228,0.373416190402291,3.93987837863393));
#8968=CARTESIAN_POINT('Ctrl Pts',(-1.09581923957444,-0.247931090158792,
3.97177133910303));
#8969=CARTESIAN_POINT('Ctrl Pts',(-0.795058502865452,-0.791907253963627,
4.00362670823387));
#8970=CARTESIAN_POINT('Ctrl Pts',(-0.251647494919828,-1.09210956787375,
4.03544259599333));
#8971=CARTESIAN_POINT('Ctrl Pts',(0.367379394643827,-1.05723105471296,4.06721734153362));
#8972=CARTESIAN_POINT('Ctrl Pts',(0.872287547395435,-0.698834410234474,
4.09894925108463));
#8973=CARTESIAN_POINT('Ctrl Pts',(1.10877998781386,-0.127551616843013,4.13063668619542));
#8974=CARTESIAN_POINT('Ctrl Pts',(1.0052446536512,0.481111111451165,4.16227808117121));
#8975=CARTESIAN_POINT('Ctrl Pts',(0.594321870531113,0.940669990088406,4.1938717879661));
#8976=CARTESIAN_POINT('Ctrl Pts',(0.0028836137700018,1.11094669369995,4.2254164735472));
#8977=CARTESIAN_POINT('Ctrl Pts',(-0.587756102544925,0.940586366285575,
4.25691019880358));
#8978=CARTESIAN_POINT('Ctrl Pts',(-0.98100418266937,0.500061769547605,4.28718787478163));
#8979=CARTESIAN_POINT('Ctrl Pts',(-1.0924189681305,-0.0518986088236793,
4.31625322570434));
#8980=CARTESIAN_POINT('Ctrl Pts',(-0.932995695727251,-0.566234439465872,
4.34411668254595));
#8981=CARTESIAN_POINT('Ctrl Pts',(-0.484070307765096,-1.00664758476799,
4.37657109924072));
#8982=CARTESIAN_POINT('Ctrl Pts',(0.251603665111017,-1.1170577608396,4.41358577518597));
#8983=CARTESIAN_POINT('Ctrl Pts',(0.942532607043053,-0.645899595864585,
4.45512260600759));
#8984=CARTESIAN_POINT('Ctrl Pts',(1.12727625401763,0.166757495434457,4.4965526452627));
#8985=CARTESIAN_POINT('Ctrl Pts',(0.711535392414827,0.886568160592581,4.53787467403547));
#8986=CARTESIAN_POINT('Ctrl Pts',(-0.0817754479350662,1.13077645625679,
4.57908545141459));
#8987=CARTESIAN_POINT('Ctrl Pts',(-0.742544779926902,0.810887680269329,
4.61561571764965));
#8988=CARTESIAN_POINT('Ctrl Pts',(-1.0367889170548,0.267632475490702,4.64750621726079));
#8989=CARTESIAN_POINT('Ctrl Pts',(-1.03661273079663,-0.259890812374001,
4.67479142272022));
#8990=CARTESIAN_POINT('Ctrl Pts',(-0.784674395084709,-0.722985135309321,
4.70202319451165));
#8991=CARTESIAN_POINT('Ctrl Pts',(-0.342665105846928,-1.0078013893598,4.72920190577311));
#8992=CARTESIAN_POINT('Ctrl Pts',(0.180728280565742,-1.04730098586176,4.75632941787614));
#8993=CARTESIAN_POINT('Ctrl Pts',(0.588474355690808,-0.862865648071463,
4.77945118635523));
#8994=CARTESIAN_POINT('Ctrl Pts',(0.837298510008721,-0.599056189202392,
4.79859890763443));
#8995=CARTESIAN_POINT('Ctrl Pts',(1.01384364614042,-0.258411401611501,4.81884983955842));
#8996=CARTESIAN_POINT('Ctrl Pts',(1.04161074189106,0.233686771419479,4.84411811105277));
#8997=CARTESIAN_POINT('Ctrl Pts',(0.755768464274831,0.75035189256676,4.87437275136583));
#8998=CARTESIAN_POINT('Ctrl Pts',(0.240260832126417,1.03503398641502,4.90455785690813));
#8999=CARTESIAN_POINT('Ctrl Pts',(-0.346443076772766,1.00191052777563,4.93467391487705));
#9000=CARTESIAN_POINT('Ctrl Pts',(-0.824443961186794,0.662491998876826,
4.96472035161675));
#9001=CARTESIAN_POINT('Ctrl Pts',(-1.04809749408919,0.122047597909646,4.99469718541711));
#9002=CARTESIAN_POINT('Ctrl Pts',(-0.950155996017736,-0.453210166677515,
5.02460427322952));
#9003=CARTESIAN_POINT('Ctrl Pts',(-0.562083374811871,-0.887170351531481,
5.05444164408033));
#9004=CARTESIAN_POINT('Ctrl Pts',(-0.00391861514886455,-1.04777194538233,
5.08420934418352));
#9005=CARTESIAN_POINT('Ctrl Pts',(0.552831610598961,-0.887172147683135,
5.11390750584928));
#9006=CARTESIAN_POINT('Ctrl Pts',(0.937898903203791,-0.455990569053019,
5.14353631321098));
#9007=CARTESIAN_POINT('Ctrl Pts',(1.03431638593341,0.112638134192545,5.17309601934115));
#9008=CARTESIAN_POINT('Ctrl Pts',(0.813941584329194,0.644164866246659,5.20258693124811));
#9009=CARTESIAN_POINT('Ctrl Pts',(0.345645707405533,0.976202338133972,5.23200943013856));
#9010=CARTESIAN_POINT('Ctrl Pts',(-0.226201062045275,1.0081223330431,5.26136393052504));
#9011=CARTESIAN_POINT('Ctrl Pts',(-0.726229018344627,0.731549687209916,
5.29065096134688));
#9012=CARTESIAN_POINT('Ctrl Pts',(-1.0018409132178,0.232472985169518,5.31987098313559));
#9013=CARTESIAN_POINT('Ctrl Pts',(-0.969765726171833,-0.335436557731811,
5.34902478961936));
#9014=CARTESIAN_POINT('Ctrl Pts',(-0.64121170398132,-0.798235214103243,
5.378112596859));
#9015=CARTESIAN_POINT('Ctrl Pts',(-0.117992925426973,-1.01474627932904,
5.40713604807643));
#9016=CARTESIAN_POINT('Ctrl Pts',(0.438971330353334,-0.9201244737966,5.43609371817436));
#9017=CARTESIAN_POINT('Ctrl Pts',(0.859207049494131,-0.544141904102835,
5.46499108972057));
#9018=CARTESIAN_POINT('Ctrl Pts',(0.962831133440289,-0.184383467346616,
5.48420765452691));
#9019=CARTESIAN_POINT('Ctrl Pts',(0.962855463572385,-0.00365305179164034,
5.49381489570681));
#9020=CARTESIAN_POINT('Ctrl Pts',(0.999999464043874,0.00398121802342207,
2.00010574185718));
#9021=CARTESIAN_POINT('Ctrl Pts',(0.999974206061282,0.19160391813607,2.01007936209659));
#9022=CARTESIAN_POINT('Ctrl Pts',(0.892358674149497,0.565284907029969,2.03003975780563));
#9023=CARTESIAN_POINT('Ctrl Pts',(0.455908354460267,0.955754980387012,2.06005123671475));
#9024=CARTESIAN_POINT('Ctrl Pts',(-0.122563158588718,1.05404138225222,2.09012808179557));
#9025=CARTESIAN_POINT('Ctrl Pts',(-0.665982422429721,0.829161410069987,
2.12027227517451));
#9026=CARTESIAN_POINT('Ctrl Pts',(-1.00720268117277,0.348508238874394,2.15048257508427));
#9027=CARTESIAN_POINT('Ctrl Pts',(-1.04050120808252,-0.241264621011279,
2.18075912672908));
#9028=CARTESIAN_POINT('Ctrl Pts',(-0.754298406118339,-0.759496345182109,
2.21110138862918));
#9029=CARTESIAN_POINT('Ctrl Pts',(-0.235139085598783,-1.04662471701868,
2.24150905560043));
#9030=CARTESIAN_POINT('Ctrl Pts',(0.358466657407177,-1.0134893307861,2.27198163744466));
#9031=CARTESIAN_POINT('Ctrl Pts',(0.844481314225998,-0.668830870873697,
2.30251864881201));
#9032=CARTESIAN_POINT('Ctrl Pts',(1.07309171546203,-0.117397710656463,2.33311952120739));
#9033=CARTESIAN_POINT('Ctrl Pts',(0.973085863935879,0.472631726678538,2.36378364003101));
#9034=CARTESIAN_POINT('Ctrl Pts',(0.640186615940372,0.844850208282888,2.38938921676183));
#9035=CARTESIAN_POINT('Ctrl Pts',(0.285207254948024,1.00321211946817,2.40990460122644));
#9036=CARTESIAN_POINT('Ctrl Pts',(-0.00357278466147455,1.04413748919053,
2.42530650345941));
#9037=CARTESIAN_POINT('Ctrl Pts',(-0.292753333069628,1.00327492007872,2.4407236705559));
#9038=CARTESIAN_POINT('Ctrl Pts',(-0.559610149845377,0.883939984413932,
2.45615599894115));
#9039=CARTESIAN_POINT('Ctrl Pts',(-0.783072629292576,0.695150535469123,
2.47160338259101));
#9040=CARTESIAN_POINT('Ctrl Pts',(-0.9883155178948,0.388599518613216,2.49107446360262));
#9041=CARTESIAN_POINT('Ctrl Pts',(-1.06097928852007,0.0299698265249316,
2.50999804459158));
#9042=CARTESIAN_POINT('Ctrl Pts',(-1.00026874085688,-0.31207309433285,2.52837129391011));
#9043=CARTESIAN_POINT('Ctrl Pts',(-0.85772117693898,-0.628943233787528,
2.54675983289627));
#9044=CARTESIAN_POINT('Ctrl Pts',(-0.539023756454129,-0.940248430945502,
2.56977396086322));
#9045=CARTESIAN_POINT('Ctrl Pts',(-0.0813539710712336,-1.06875629404709,
2.59436218564022));
#9046=CARTESIAN_POINT('Ctrl Pts',(0.440709506996878,-0.995074461032676,
2.6220606386953));
#9047=CARTESIAN_POINT('Ctrl Pts',(0.881652173543376,-0.668351901468915,
2.64980261114177));
#9048=CARTESIAN_POINT('Ctrl Pts',(1.0852948664173,-0.105373203004237,2.68068203601616));
#9049=CARTESIAN_POINT('Ctrl Pts',(1.00539530848997,0.426480980519131,2.70851510392812));
#9050=CARTESIAN_POINT('Ctrl Pts',(0.679609573339881,0.857002336026301,2.7363888804944));
#9051=CARTESIAN_POINT('Ctrl Pts',(0.242228396206659,1.05406947259606,2.76120094819001));
#9052=CARTESIAN_POINT('Ctrl Pts',(-0.289433825273236,1.05900157503401,2.78914691397882));
#9053=CARTESIAN_POINT('Ctrl Pts',(-0.861030373991185,0.756502517113054,
2.82179513727801));
#9054=CARTESIAN_POINT('Ctrl Pts',(-1.15948386741598,-0.00245881106342116,
2.8622922968233));
#9055=CARTESIAN_POINT('Ctrl Pts',(-0.849819252545902,-0.791606149879273,
2.9044266522989));
#9056=CARTESIAN_POINT('Ctrl Pts',(-0.0848273064559805,-1.16047682132822,
2.94663705560064));
#9057=CARTESIAN_POINT('Ctrl Pts',(0.728338616139595,-0.909963609903424,
2.98891980674896));
#9058=CARTESIAN_POINT('Ctrl Pts',(1.15452570093491,-0.172022292800125,3.03127110274204));
#9059=CARTESIAN_POINT('Ctrl Pts',(0.965079959728901,0.659906484623926,3.07368702284038));
#9060=CARTESIAN_POINT('Ctrl Pts',(0.258512451458961,1.14196808324737,3.11616354351132));
#9061=CARTESIAN_POINT('Ctrl Pts',(-0.492717397384934,1.02781794268986,3.15397066853381));
#9062=CARTESIAN_POINT('Ctrl Pts',(-0.950847731766782,0.578891230696036,
3.18708578741999));
#9063=CARTESIAN_POINT('Ctrl Pts',(-1.11322603418831,0.0543699563964829,
3.21549214280387));
#9064=CARTESIAN_POINT('Ctrl Pts',(-1.00397682800075,-0.485299668185688,
3.24391918371992));
#9065=CARTESIAN_POINT('Ctrl Pts',(-0.689560596566738,-0.85912025786842,
3.2692049003822));
#9066=CARTESIAN_POINT('Ctrl Pts',(-0.203462101275883,-1.09903917913844,
3.29766639858301));
#9067=CARTESIAN_POINT('Ctrl Pts',(0.296274556510708,-1.07870085350966,3.32298079518316));
#9068=CARTESIAN_POINT('Ctrl Pts',(0.813909810244539,-0.768416856681802,
3.35464092662437));
#9069=CARTESIAN_POINT('Ctrl Pts',(1.10016251506307,-0.282678926353398,3.38314956983213));
#9070=CARTESIAN_POINT('Ctrl Pts',(1.06842542005047,0.330699838209083,3.41484232929802));
#9071=CARTESIAN_POINT('Ctrl Pts',(0.781036889262004,0.801635745996559,3.44337716794684));
#9072=CARTESIAN_POINT('Ctrl Pts',(0.3026681656048,1.07751158150631,3.47192198965488));
#9073=CARTESIAN_POINT('Ctrl Pts',(-0.341977208139237,1.09513778685306,3.5052343169007));
#9074=CARTESIAN_POINT('Ctrl Pts',(-0.975597618652369,0.664760099314692,
3.54331757606612));
#9075=CARTESIAN_POINT('Ctrl Pts',(-1.13429370842399,-0.0357778387848846,
3.57903024860792));
#9076=CARTESIAN_POINT('Ctrl Pts',(-0.952497172320662,-0.550291907933128,
3.60760379990449));
#9077=CARTESIAN_POINT('Ctrl Pts',(-0.68624513734708,-0.860512981218381,
3.62903507783467));
#9078=CARTESIAN_POINT('Ctrl Pts',(-0.324306798008731,-1.0514860754467,3.65046688028005));
#9079=CARTESIAN_POINT('Ctrl Pts',(0.127344232453658,-1.10276625857497,3.674279919598));
#9080=CARTESIAN_POINT('Ctrl Pts',(0.607784221866902,-0.941400265606059,
3.70047332316486));
#9081=CARTESIAN_POINT('Ctrl Pts',(0.983690388895233,-0.535896868540009,
3.72904537472281));
#9082=CARTESIAN_POINT('Ctrl Pts',(1.08731538430027,-0.128732018548745,3.75076902067426));
#9083=CARTESIAN_POINT('Ctrl Pts',(1.06753777509939,0.150334725456009,3.7656464393213));
#9084=CARTESIAN_POINT('Ctrl Pts',(1.02549367550628,0.347236435696266,3.7763575734054));
#9085=CARTESIAN_POINT('Ctrl Pts',(0.880884191480398,0.671592660752369,3.7951003560531));
#9086=CARTESIAN_POINT('Ctrl Pts',(0.491799935626419,1.0196644890383,3.82187027476111));
#9087=CARTESIAN_POINT('Ctrl Pts',(-0.126065746592581,1.12455786056488,3.85398342973913));
#9088=CARTESIAN_POINT('Ctrl Pts',(-0.704583522010695,0.88486307777345,3.88608387297236));
#9089=CARTESIAN_POINT('Ctrl Pts',(-1.06683466983354,0.3742832244399,3.91816964977168));
#9090=CARTESIAN_POINT('Ctrl Pts',(-1.10184933977514,-0.250419432627018,
3.95023881727803));
#9091=CARTESIAN_POINT('Ctrl Pts',(-0.799326718711519,-0.797694380880393,
3.98228945733906));
#9092=CARTESIAN_POINT('Ctrl Pts',(-0.252343111177166,-1.09993153075449,
4.01431965364637));
#9093=CARTESIAN_POINT('Ctrl Pts',(0.371159169345164,-1.06485412373635,4.0463275194738));
#9094=CARTESIAN_POINT('Ctrl Pts',(0.880047504125487,-0.703696890362346,
4.07831118189475));
#9095=CARTESIAN_POINT('Ctrl Pts',(1.11857837754389,-0.127626743256515,4.11026879475596));
#9096=CARTESIAN_POINT('Ctrl Pts',(1.01416153614381,0.486524030990474,4.14219853012843));
#9097=CARTESIAN_POINT('Ctrl Pts',(0.599338058827864,0.950520440175857,4.17409858361638));
#9098=CARTESIAN_POINT('Ctrl Pts',(0.00190308953361062,1.12257447034417,
4.20596718959497));
#9099=CARTESIAN_POINT('Ctrl Pts',(-0.595087816877256,0.950429978912684,
4.23780259148061));
#9100=CARTESIAN_POINT('Ctrl Pts',(-0.992818074176864,0.504960206465758,
4.26842528448615));
#9101=CARTESIAN_POINT('Ctrl Pts',(-1.10558192615926,-0.0535255134762696,
4.29783816996833));
#9102=CARTESIAN_POINT('Ctrl Pts',(-0.944245633155887,-0.574182433998452,
4.326044460862));
#9103=CARTESIAN_POINT('Ctrl Pts',(-0.489615552103502,-1.02023046107543,
4.35891537170686));
#9104=CARTESIAN_POINT('Ctrl Pts',(0.255873406558148,-1.13223620757883,4.39642822383059));
#9105=CARTESIAN_POINT('Ctrl Pts',(0.956585537399415,-0.654531370431507,
4.43855371945495));
#9106=CARTESIAN_POINT('Ctrl Pts',(1.14416456861692,0.170066871142059,4.48059920430672));
#9107=CARTESIAN_POINT('Ctrl Pts',(0.722117099067864,0.901002181388938,4.52256123999552));
#9108=CARTESIAN_POINT('Ctrl Pts',(-0.0838676738781217,1.14921441407926,
4.5644365266184));
#9109=CARTESIAN_POINT('Ctrl Pts',(-0.755677502986392,0.824069849946143,
4.60157908243497));
#9110=CARTESIAN_POINT('Ctrl Pts',(-1.05498104408691,0.271521112381307,4.63401858831428));
#9111=CARTESIAN_POINT('Ctrl Pts',(-1.05483403133078,-0.26522135570406,4.66178172056988));
#9112=CARTESIAN_POINT('Ctrl Pts',(-0.79840547489227,-0.736599185468657,
4.68950186792131));
#9113=CARTESIAN_POINT('Ctrl Pts',(-0.3483499377511,-1.02663834291108,4.71717822726345));
#9114=CARTESIAN_POINT('Ctrl Pts',(0.184757632451299,-1.06688722115596,4.74481003558103));
#9115=CARTESIAN_POINT('Ctrl Pts',(0.600256695779753,-0.878980608467174,
4.7683735201888));
#9116=CARTESIAN_POINT('Ctrl Pts',(0.853850233649786,-0.610120445383555,
4.78788851920089));
#9117=CARTESIAN_POINT('Ctrl Pts',(1.03381570897682,-0.262894148472765,4.80853189587555));
#9118=CARTESIAN_POINT('Ctrl Pts',(1.06215687349528,0.238874309450968,4.83429913779336));
#9119=CARTESIAN_POINT('Ctrl Pts',(0.770634803840811,0.765869068483215,4.86515976481244));
#9120=CARTESIAN_POINT('Ctrl Pts',(0.244684747552399,1.05635550605388,4.89595947659513));
#9121=CARTESIAN_POINT('Ctrl Pts',(-0.354100647382748,1.02257824395859,4.92669748292077));
#9122=CARTESIAN_POINT('Ctrl Pts',(-0.842095960257555,0.676096127224308,
4.95737304397893));
#9123=CARTESIAN_POINT('Ctrl Pts',(-1.07050216965279,0.124232350128257,4.98798547954758));
#9124=CARTESIAN_POINT('Ctrl Pts',(-0.970487698233666,-0.463339790807337,
5.01853416178037));
#9125=CARTESIAN_POINT('Ctrl Pts',(-0.57403535125674,-0.906703305752076,
5.04901852189829));
#9126=CARTESIAN_POINT('Ctrl Pts',(-0.00367933936324437,-1.07083384017741,
5.07943804916124));
#9127=CARTESIAN_POINT('Ctrl Pts',(0.56535226719551,-0.906710964597204,5.10979228847672));
#9128=CARTESIAN_POINT('Ctrl Pts',(0.95899197878984,-0.465956326824321,5.14008084401914));
#9129=CARTESIAN_POINT('Ctrl Pts',(1.05758360680831,0.115400410376887,5.17030337915801));
#9130=CARTESIAN_POINT('Ctrl Pts',(0.832257130959616,0.658907139635372,5.20045961311858));
#9131=CARTESIAN_POINT('Ctrl Pts',(0.353362036446966,0.998475173781019,5.23054933034559));
#9132=CARTESIAN_POINT('Ctrl Pts',(-0.231493376683462,1.03113233690688,5.26057235733975));
#9133=CARTESIAN_POINT('Ctrl Pts',(-0.742941371583914,0.748253733713579,
5.29052861685377));
#9134=CARTESIAN_POINT('Ctrl Pts',(-1.02486870130036,0.23775759542928,5.3204180022368));
#9135=CARTESIAN_POINT('Ctrl Pts',(-0.992064317380329,-0.343173817499407,
5.3502406538254));
#9136=CARTESIAN_POINT('Ctrl Pts',(-0.655975229859479,-0.81659286891466,
5.37999633599993));
#9137=CARTESIAN_POINT('Ctrl Pts',(-0.120753665413257,-1.03807600951265,
5.40968580999697));
#9138=CARTESIAN_POINT('Ctrl Pts',(0.44897427078276,-0.941278849111864,5.43930775328404));
#9139=CARTESIAN_POINT('Ctrl Pts',(0.878820594563222,-0.556707495126734,
5.46886560818098));
#9140=CARTESIAN_POINT('Ctrl Pts',(0.984806813297395,-0.188706783169536,
5.48852259094232));
#9141=CARTESIAN_POINT('Ctrl Pts',(0.984831692610592,-0.00389691057600537,
5.49834668730695));
#9142=CARTESIAN_POINT('',(0.999999464043874,0.00398121802342206,2.00010574185718));
#9143=CARTESIAN_POINT('Origin',(1.,0.,2.075));
#9144=CARTESIAN_POINT('',(0.984831692610592,-0.00389691057600538,5.49834668730695));
#9145=CARTESIAN_POINT('Ctrl Pts',(0.999999464043874,0.00398121802342207,
2.00010574185718));
#9146=CARTESIAN_POINT('Ctrl Pts',(0.999974206061282,0.19160391813607,2.01007936209659));
#9147=CARTESIAN_POINT('Ctrl Pts',(0.892358674149497,0.565284907029969,2.03003975780563));
#9148=CARTESIAN_POINT('Ctrl Pts',(0.455908354460267,0.955754980387012,2.06005123671475));
#9149=CARTESIAN_POINT('Ctrl Pts',(-0.122563158588718,1.05404138225222,2.09012808179557));
#9150=CARTESIAN_POINT('Ctrl Pts',(-0.665982422429721,0.829161410069987,
2.12027227517451));
#9151=CARTESIAN_POINT('Ctrl Pts',(-1.00720268117277,0.348508238874394,2.15048257508427));
#9152=CARTESIAN_POINT('Ctrl Pts',(-1.04050120808252,-0.241264621011279,
2.18075912672908));
#9153=CARTESIAN_POINT('Ctrl Pts',(-0.754298406118339,-0.759496345182109,
2.21110138862918));
#9154=CARTESIAN_POINT('Ctrl Pts',(-0.235139085598783,-1.04662471701868,
2.24150905560043));
#9155=CARTESIAN_POINT('Ctrl Pts',(0.358466657407177,-1.0134893307861,2.27198163744466));
#9156=CARTESIAN_POINT('Ctrl Pts',(0.844481314225998,-0.668830870873697,
2.30251864881201));
#9157=CARTESIAN_POINT('Ctrl Pts',(1.07309171546203,-0.117397710656463,2.33311952120739));
#9158=CARTESIAN_POINT('Ctrl Pts',(0.973085863935879,0.472631726678538,2.36378364003101));
#9159=CARTESIAN_POINT('Ctrl Pts',(0.640186615940372,0.844850208282888,2.38938921676183));
#9160=CARTESIAN_POINT('Ctrl Pts',(0.285207254948024,1.00321211946817,2.40990460122644));
#9161=CARTESIAN_POINT('Ctrl Pts',(-0.00357278466147455,1.04413748919053,
2.42530650345941));
#9162=CARTESIAN_POINT('Ctrl Pts',(-0.292753333069628,1.00327492007872,2.4407236705559));
#9163=CARTESIAN_POINT('Ctrl Pts',(-0.559610149845377,0.883939984413932,
2.45615599894115));
#9164=CARTESIAN_POINT('Ctrl Pts',(-0.783072629292576,0.695150535469123,
2.47160338259101));
#9165=CARTESIAN_POINT('Ctrl Pts',(-0.9883155178948,0.388599518613216,2.49107446360262));
#9166=CARTESIAN_POINT('Ctrl Pts',(-1.06097928852007,0.0299698265249316,
2.50999804459158));
#9167=CARTESIAN_POINT('Ctrl Pts',(-1.00026874085688,-0.31207309433285,2.52837129391011));
#9168=CARTESIAN_POINT('Ctrl Pts',(-0.85772117693898,-0.628943233787528,
2.54675983289627));
#9169=CARTESIAN_POINT('Ctrl Pts',(-0.539023756454129,-0.940248430945502,
2.56977396086322));
#9170=CARTESIAN_POINT('Ctrl Pts',(-0.0813539710712336,-1.06875629404709,
2.59436218564022));
#9171=CARTESIAN_POINT('Ctrl Pts',(0.440709506996878,-0.995074461032676,
2.6220606386953));
#9172=CARTESIAN_POINT('Ctrl Pts',(0.881652173543376,-0.668351901468915,
2.64980261114177));
#9173=CARTESIAN_POINT('Ctrl Pts',(1.0852948664173,-0.105373203004237,2.68068203601616));
#9174=CARTESIAN_POINT('Ctrl Pts',(1.00539530848997,0.426480980519131,2.70851510392812));
#9175=CARTESIAN_POINT('Ctrl Pts',(0.679609573339881,0.857002336026301,2.7363888804944));
#9176=CARTESIAN_POINT('Ctrl Pts',(0.242228396206659,1.05406947259606,2.76120094819001));
#9177=CARTESIAN_POINT('Ctrl Pts',(-0.289433825273236,1.05900157503401,2.78914691397882));
#9178=CARTESIAN_POINT('Ctrl Pts',(-0.861030373991185,0.756502517113054,
2.82179513727801));
#9179=CARTESIAN_POINT('Ctrl Pts',(-1.15948386741598,-0.00245881106342116,
2.8622922968233));
#9180=CARTESIAN_POINT('Ctrl Pts',(-0.849819252545902,-0.791606149879273,
2.9044266522989));
#9181=CARTESIAN_POINT('Ctrl Pts',(-0.0848273064559805,-1.16047682132822,
2.94663705560064));
#9182=CARTESIAN_POINT('Ctrl Pts',(0.728338616139595,-0.909963609903424,
2.98891980674896));
#9183=CARTESIAN_POINT('Ctrl Pts',(1.15452570093491,-0.172022292800125,3.03127110274204));
#9184=CARTESIAN_POINT('Ctrl Pts',(0.965079959728901,0.659906484623926,3.07368702284038));
#9185=CARTESIAN_POINT('Ctrl Pts',(0.258512451458961,1.14196808324737,3.11616354351132));
#9186=CARTESIAN_POINT('Ctrl Pts',(-0.492717397384934,1.02781794268986,3.15397066853381));
#9187=CARTESIAN_POINT('Ctrl Pts',(-0.950847731766782,0.578891230696036,
3.18708578741999));
#9188=CARTESIAN_POINT('Ctrl Pts',(-1.11322603418831,0.0543699563964829,
3.21549214280387));
#9189=CARTESIAN_POINT('Ctrl Pts',(-1.00397682800075,-0.485299668185688,
3.24391918371992));
#9190=CARTESIAN_POINT('Ctrl Pts',(-0.689560596566738,-0.85912025786842,
3.2692049003822));
#9191=CARTESIAN_POINT('Ctrl Pts',(-0.203462101275883,-1.09903917913844,
3.29766639858301));
#9192=CARTESIAN_POINT('Ctrl Pts',(0.296274556510708,-1.07870085350966,3.32298079518316));
#9193=CARTESIAN_POINT('Ctrl Pts',(0.813909810244539,-0.768416856681802,
3.35464092662437));
#9194=CARTESIAN_POINT('Ctrl Pts',(1.10016251506307,-0.282678926353398,3.38314956983213));
#9195=CARTESIAN_POINT('Ctrl Pts',(1.06842542005047,0.330699838209083,3.41484232929802));
#9196=CARTESIAN_POINT('Ctrl Pts',(0.781036889262004,0.801635745996559,3.44337716794684));
#9197=CARTESIAN_POINT('Ctrl Pts',(0.3026681656048,1.07751158150631,3.47192198965488));
#9198=CARTESIAN_POINT('Ctrl Pts',(-0.341977208139237,1.09513778685306,3.5052343169007));
#9199=CARTESIAN_POINT('Ctrl Pts',(-0.975597618652369,0.664760099314692,
3.54331757606612));
#9200=CARTESIAN_POINT('Ctrl Pts',(-1.13429370842399,-0.0357778387848846,
3.57903024860792));
#9201=CARTESIAN_POINT('Ctrl Pts',(-0.952497172320662,-0.550291907933128,
3.60760379990449));
#9202=CARTESIAN_POINT('Ctrl Pts',(-0.68624513734708,-0.860512981218381,
3.62903507783467));
#9203=CARTESIAN_POINT('Ctrl Pts',(-0.324306798008731,-1.0514860754467,3.65046688028005));
#9204=CARTESIAN_POINT('Ctrl Pts',(0.127344232453658,-1.10276625857497,3.674279919598));
#9205=CARTESIAN_POINT('Ctrl Pts',(0.607784221866902,-0.941400265606059,
3.70047332316486));
#9206=CARTESIAN_POINT('Ctrl Pts',(0.983690388895233,-0.535896868540009,
3.72904537472281));
#9207=CARTESIAN_POINT('Ctrl Pts',(1.08731538430027,-0.128732018548745,3.75076902067426));
#9208=CARTESIAN_POINT('Ctrl Pts',(1.06753777509939,0.150334725456009,3.7656464393213));
#9209=CARTESIAN_POINT('Ctrl Pts',(1.02549367550628,0.347236435696266,3.7763575734054));
#9210=CARTESIAN_POINT('Ctrl Pts',(0.880884191480398,0.671592660752369,3.7951003560531));
#9211=CARTESIAN_POINT('Ctrl Pts',(0.491799935626419,1.0196644890383,3.82187027476111));
#9212=CARTESIAN_POINT('Ctrl Pts',(-0.126065746592581,1.12455786056488,3.85398342973913));
#9213=CARTESIAN_POINT('Ctrl Pts',(-0.704583522010695,0.88486307777345,3.88608387297236));
#9214=CARTESIAN_POINT('Ctrl Pts',(-1.06683466983354,0.3742832244399,3.91816964977168));
#9215=CARTESIAN_POINT('Ctrl Pts',(-1.10184933977514,-0.250419432627018,
3.95023881727803));
#9216=CARTESIAN_POINT('Ctrl Pts',(-0.799326718711519,-0.797694380880393,
3.98228945733906));
#9217=CARTESIAN_POINT('Ctrl Pts',(-0.252343111177166,-1.09993153075449,
4.01431965364637));
#9218=CARTESIAN_POINT('Ctrl Pts',(0.371159169345164,-1.06485412373635,4.0463275194738));
#9219=CARTESIAN_POINT('Ctrl Pts',(0.880047504125487,-0.703696890362346,
4.07831118189475));
#9220=CARTESIAN_POINT('Ctrl Pts',(1.11857837754389,-0.127626743256515,4.11026879475596));
#9221=CARTESIAN_POINT('Ctrl Pts',(1.01416153614381,0.486524030990474,4.14219853012843));
#9222=CARTESIAN_POINT('Ctrl Pts',(0.599338058827864,0.950520440175857,4.17409858361638));
#9223=CARTESIAN_POINT('Ctrl Pts',(0.00190308953361062,1.12257447034417,
4.20596718959497));
#9224=CARTESIAN_POINT('Ctrl Pts',(-0.595087816877256,0.950429978912684,
4.23780259148061));
#9225=CARTESIAN_POINT('Ctrl Pts',(-0.992818074176864,0.504960206465758,
4.26842528448615));
#9226=CARTESIAN_POINT('Ctrl Pts',(-1.10558192615926,-0.0535255134762696,
4.29783816996833));
#9227=CARTESIAN_POINT('Ctrl Pts',(-0.944245633155887,-0.574182433998452,
4.326044460862));
#9228=CARTESIAN_POINT('Ctrl Pts',(-0.489615552103502,-1.02023046107543,
4.35891537170686));
#9229=CARTESIAN_POINT('Ctrl Pts',(0.255873406558148,-1.13223620757883,4.39642822383059));
#9230=CARTESIAN_POINT('Ctrl Pts',(0.956585537399415,-0.654531370431507,
4.43855371945495));
#9231=CARTESIAN_POINT('Ctrl Pts',(1.14416456861692,0.170066871142059,4.48059920430672));
#9232=CARTESIAN_POINT('Ctrl Pts',(0.722117099067864,0.901002181388938,4.52256123999552));
#9233=CARTESIAN_POINT('Ctrl Pts',(-0.0838676738781217,1.14921441407926,
4.5644365266184));
#9234=CARTESIAN_POINT('Ctrl Pts',(-0.755677502986392,0.824069849946143,
4.60157908243497));
#9235=CARTESIAN_POINT('Ctrl Pts',(-1.05498104408691,0.271521112381307,4.63401858831428));
#9236=CARTESIAN_POINT('Ctrl Pts',(-1.05483403133078,-0.26522135570406,4.66178172056988));
#9237=CARTESIAN_POINT('Ctrl Pts',(-0.79840547489227,-0.736599185468657,
4.68950186792131));
#9238=CARTESIAN_POINT('Ctrl Pts',(-0.3483499377511,-1.02663834291108,4.71717822726345));
#9239=CARTESIAN_POINT('Ctrl Pts',(0.184757632451299,-1.06688722115596,4.74481003558103));
#9240=CARTESIAN_POINT('Ctrl Pts',(0.600256695779753,-0.878980608467174,
4.7683735201888));
#9241=CARTESIAN_POINT('Ctrl Pts',(0.853850233649786,-0.610120445383555,
4.78788851920089));
#9242=CARTESIAN_POINT('Ctrl Pts',(1.03381570897682,-0.262894148472765,4.80853189587555));
#9243=CARTESIAN_POINT('Ctrl Pts',(1.06215687349528,0.238874309450968,4.83429913779336));
#9244=CARTESIAN_POINT('Ctrl Pts',(0.770634803840811,0.765869068483215,4.86515976481244));
#9245=CARTESIAN_POINT('Ctrl Pts',(0.244684747552399,1.05635550605388,4.89595947659513));
#9246=CARTESIAN_POINT('Ctrl Pts',(-0.354100647382748,1.02257824395859,4.92669748292077));
#9247=CARTESIAN_POINT('Ctrl Pts',(-0.842095960257555,0.676096127224308,
4.95737304397893));
#9248=CARTESIAN_POINT('Ctrl Pts',(-1.07050216965279,0.124232350128257,4.98798547954758));
#9249=CARTESIAN_POINT('Ctrl Pts',(-0.970487698233666,-0.463339790807337,
5.01853416178037));
#9250=CARTESIAN_POINT('Ctrl Pts',(-0.57403535125674,-0.906703305752076,
5.04901852189829));
#9251=CARTESIAN_POINT('Ctrl Pts',(-0.00367933936324437,-1.07083384017741,
5.07943804916124));
#9252=CARTESIAN_POINT('Ctrl Pts',(0.56535226719551,-0.906710964597204,5.10979228847672));
#9253=CARTESIAN_POINT('Ctrl Pts',(0.95899197878984,-0.465956326824321,5.14008084401914));
#9254=CARTESIAN_POINT('Ctrl Pts',(1.05758360680831,0.115400410376887,5.17030337915801));
#9255=CARTESIAN_POINT('Ctrl Pts',(0.832257130959616,0.658907139635372,5.20045961311858));
#9256=CARTESIAN_POINT('Ctrl Pts',(0.353362036446966,0.998475173781019,5.23054933034559));
#9257=CARTESIAN_POINT('Ctrl Pts',(-0.231493376683462,1.03113233690688,5.26057235733975));
#9258=CARTESIAN_POINT('Ctrl Pts',(-0.742941371583914,0.748253733713579,
5.29052861685377));
#9259=CARTESIAN_POINT('Ctrl Pts',(-1.02486870130036,0.23775759542928,5.3204180022368));
#9260=CARTESIAN_POINT('Ctrl Pts',(-0.992064317380329,-0.343173817499407,
5.3502406538254));
#9261=CARTESIAN_POINT('Ctrl Pts',(-0.655975229859479,-0.81659286891466,
5.37999633599993));
#9262=CARTESIAN_POINT('Ctrl Pts',(-0.120753665413257,-1.03807600951265,
5.40968580999697));
#9263=CARTESIAN_POINT('Ctrl Pts',(0.44897427078276,-0.941278849111864,5.43930775328404));
#9264=CARTESIAN_POINT('Ctrl Pts',(0.878820594563222,-0.556707495126734,
5.46886560818098));
#9265=CARTESIAN_POINT('Ctrl Pts',(0.984806813297395,-0.188706783169536,
5.48852259094232));
#9266=CARTESIAN_POINT('Ctrl Pts',(0.984831692610592,-0.00389691057600537,
5.49834668730695));
#9267=CARTESIAN_POINT('Origin',(1.,-2.44249065417534E-15,5.425));
#9268=CARTESIAN_POINT('Origin',(1.,-2.44249065417534E-15,5.425));
#9269=CARTESIAN_POINT('Origin',(1.,0.,2.075));
#10571=UNCERTAINTY_MEASURE_WITH_UNIT(LENGTH_MEASURE(0.001),#10628,
'DISTANCE_ACCURACY_VALUE',
'Maximum model space distance between geometric entities at asserted c
onnectivities');
#10595=UNCERTAINTY_MEASURE_WITH_UNIT(LENGTH_MEASURE(0.001),#10628,
'DISTANCE_ACCURACY_VALUE',
'Maximum model space distance between geometric entities at asserted c
onnectivities');
#10603=(
GEOMETRIC_REPRESENTATION_CONTEXT(3)
GLOBAL_UNCERTAINTY_ASSIGNED_CONTEXT((#10571))
GLOBAL_UNIT_ASSIGNED_CONTEXT((#10628,#10630,#10631))
REPRESENTATION_CONTEXT('','3D')
);
#10627=(
GEOMETRIC_REPRESENTATION_CONTEXT(3)
GLOBAL_UNCERTAINTY_ASSIGNED_CONTEXT((#10595))
GLOBAL_UNIT_ASSIGNED_CONTEXT((#10628,#10630,#10631))
REPRESENTATION_CONTEXT('','3D')
);
#10628=(
LENGTH_UNIT()
NAMED_UNIT(*)
SI_UNIT(.CENTI.,.METRE.)
);
#10630=(
NAMED_UNIT(*)
PLANE_ANGLE_UNIT()
SI_UNIT($,.RADIAN.)
);
#10631=(
NAMED_UNIT(*)
SI_UNIT($,.STERADIAN.)
SOLID_ANGLE_UNIT()
);
#10639=SHAPE_DEFINITION_REPRESENTATION(#10670,#10744);
#10670=PRODUCT_DEFINITION_SHAPE('',$,#10776);
#10744=SHAPE_REPRESENTATION('',(#5366),#10603);
#10768=PRODUCT_DEFINITION_CONTEXT('part definition',#10863,'design');
#10776=PRODUCT_DEFINITION('Installed lift spring',
'Installed lift spring',#10807,#10768);
#10807=PRODUCT_DEFINITION_FORMATION('',$,#10872);
#10863=APPLICATION_CONTEXT(
'Core Data for Automotive Mechanical Design Process');
#10864=PRODUCT_CONTEXT('part definition',#10863,'mechanical');
#10872=PRODUCT('Installed lift spring','Installed lift spring',
'Installed lift spring',(#10864));
#10959=COLOUR_RGB('Grey',0.48,0.52,0.57);
#10960=FILL_AREA_STYLE_COLOUR('',#10959);
#10961=FILL_AREA_STYLE('',(#10960));
#10962=SURFACE_STYLE_FILL_AREA(#10961);
#10963=SURFACE_SIDE_STYLE('',(#10962));
#10964=SURFACE_STYLE_USAGE(.BOTH.,#10963);
#10965=PRESENTATION_STYLE_ASSIGNMENT((#10964));
ENDSEC;
END-ISO-10303-21;
